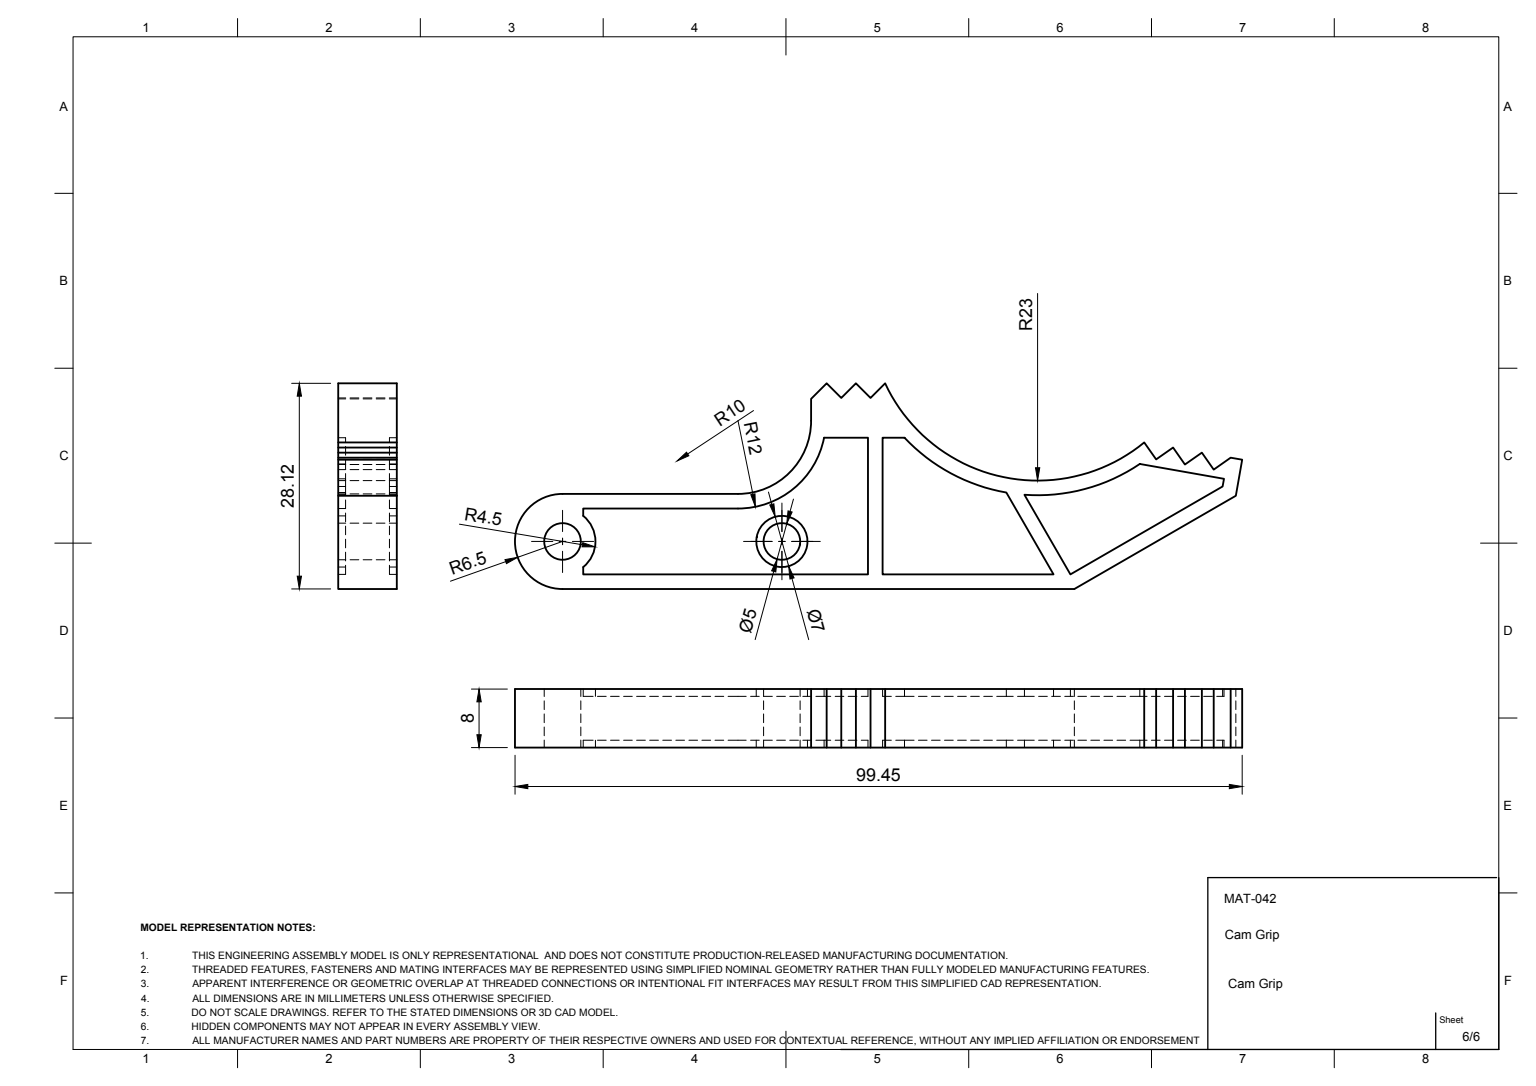
ISO-10303-21;
HEADER;
/* Generated by software containing ST-Developer
 * from STEP Tools, Inc. (www.steptools.com) 
 */

FILE_DESCRIPTION(
/* description */ ('STEP AP214'),
/* implementation_level */ '2;1');

FILE_NAME(
/* name */ 'Cam Grip.step',
/* time_stamp */ '2026-11-14T22:03:06-08:00',
/* author */ (''),
/* organization */ (''),
/* preprocessor_version */ 'ST-DEVELOPER v20.2',
/* originating_system */ 'Autodesk Translation Framework v15.17.0.0',
/* authorisation */ '');

FILE_SCHEMA (('AUTOMOTIVE_DESIGN { 1 0 10303 214 3 1 1 }'));
ENDSEC;

DATA;
#10=MECHANICAL_DESIGN_GEOMETRIC_PRESENTATION_REPRESENTATION('',(#308),#12966);
#288=SHAPE_REPRESENTATION_RELATIONSHIP('SRR','None',#13026,#296);
#296=ADVANCED_BREP_SHAPE_REPRESENTATION('',(#320),#12959);
#308=STYLED_ITEM('',(#13075),#320);
#320=MANIFOLD_SOLID_BREP('Body1',#5583);
#355=FACE_BOUND('',#953,.T.);
#356=FACE_BOUND('',#955,.T.);
#357=FACE_BOUND('',#957,.T.);
#358=FACE_BOUND('',#958,.T.);
#359=FACE_BOUND('',#959,.T.);
#360=FACE_BOUND('',#960,.T.);
#361=FACE_BOUND('',#962,.T.);
#362=FACE_BOUND('',#963,.T.);
#363=FACE_BOUND('',#964,.T.);
#364=FACE_BOUND('',#965,.T.);
#365=FACE_BOUND('',#1007,.T.);
#366=FACE_BOUND('',#1016,.T.);
#425=PLANE('',#5799);
#426=PLANE('',#5800);
#427=PLANE('',#5801);
#428=PLANE('',#5809);
#429=PLANE('',#5816);
#430=PLANE('',#5817);
#431=PLANE('',#5819);
#432=PLANE('',#5821);
#433=PLANE('',#5822);
#434=PLANE('',#5823);
#435=PLANE('',#5824);
#436=PLANE('',#5825);
#437=PLANE('',#5826);
#438=PLANE('',#5828);
#439=PLANE('',#5829);
#440=PLANE('',#5830);
#441=PLANE('',#5831);
#442=PLANE('',#5832);
#443=PLANE('',#5833);
#444=PLANE('',#5834);
#445=PLANE('',#5835);
#446=PLANE('',#5836);
#447=PLANE('',#5837);
#448=PLANE('',#5838);
#449=PLANE('',#5839);
#450=PLANE('',#5842);
#451=PLANE('',#5843);
#452=PLANE('',#5844);
#453=PLANE('',#5845);
#454=PLANE('',#5848);
#455=PLANE('',#5849);
#456=PLANE('',#5852);
#457=PLANE('',#5853);
#458=PLANE('',#5854);
#459=PLANE('',#5855);
#460=PLANE('',#5858);
#461=PLANE('',#5859);
#462=PLANE('',#5860);
#463=PLANE('',#5861);
#464=PLANE('',#5862);
#465=PLANE('',#5865);
#466=PLANE('',#5866);
#467=PLANE('',#5867);
#468=PLANE('',#5868);
#469=PLANE('',#5869);
#470=PLANE('',#5870);
#471=PLANE('',#5871);
#472=PLANE('',#5874);
#473=PLANE('',#5875);
#474=PLANE('',#5876);
#475=PLANE('',#5877);
#476=PLANE('',#5878);
#477=PLANE('',#5879);
#478=PLANE('',#5882);
#479=PLANE('',#5883);
#608=FACE_OUTER_BOUND('',#947,.T.);
#609=FACE_OUTER_BOUND('',#948,.T.);
#610=FACE_OUTER_BOUND('',#949,.T.);
#611=FACE_OUTER_BOUND('',#950,.T.);
#612=FACE_OUTER_BOUND('',#951,.T.);
#613=FACE_OUTER_BOUND('',#952,.T.);
#614=FACE_OUTER_BOUND('',#954,.T.);
#615=FACE_OUTER_BOUND('',#956,.T.);
#616=FACE_OUTER_BOUND('',#961,.T.);
#617=FACE_OUTER_BOUND('',#966,.T.);
#618=FACE_OUTER_BOUND('',#967,.T.);
#619=FACE_OUTER_BOUND('',#968,.T.);
#620=FACE_OUTER_BOUND('',#969,.T.);
#621=FACE_OUTER_BOUND('',#970,.T.);
#622=FACE_OUTER_BOUND('',#971,.T.);
#623=FACE_OUTER_BOUND('',#972,.T.);
#624=FACE_OUTER_BOUND('',#973,.T.);
#625=FACE_OUTER_BOUND('',#974,.T.);
#626=FACE_OUTER_BOUND('',#975,.T.);
#627=FACE_OUTER_BOUND('',#976,.T.);
#628=FACE_OUTER_BOUND('',#977,.T.);
#629=FACE_OUTER_BOUND('',#978,.T.);
#630=FACE_OUTER_BOUND('',#979,.T.);
#631=FACE_OUTER_BOUND('',#980,.T.);
#632=FACE_OUTER_BOUND('',#981,.T.);
#633=FACE_OUTER_BOUND('',#982,.T.);
#634=FACE_OUTER_BOUND('',#983,.T.);
#635=FACE_OUTER_BOUND('',#984,.T.);
#636=FACE_OUTER_BOUND('',#985,.T.);
#637=FACE_OUTER_BOUND('',#986,.T.);
#638=FACE_OUTER_BOUND('',#987,.T.);
#639=FACE_OUTER_BOUND('',#988,.T.);
#640=FACE_OUTER_BOUND('',#989,.T.);
#641=FACE_OUTER_BOUND('',#990,.T.);
#642=FACE_OUTER_BOUND('',#991,.T.);
#643=FACE_OUTER_BOUND('',#992,.T.);
#644=FACE_OUTER_BOUND('',#993,.T.);
#645=FACE_OUTER_BOUND('',#994,.T.);
#646=FACE_OUTER_BOUND('',#995,.T.);
#647=FACE_OUTER_BOUND('',#996,.T.);
#648=FACE_OUTER_BOUND('',#997,.T.);
#649=FACE_OUTER_BOUND('',#998,.T.);
#650=FACE_OUTER_BOUND('',#999,.T.);
#651=FACE_OUTER_BOUND('',#1000,.T.);
#652=FACE_OUTER_BOUND('',#1001,.T.);
#653=FACE_OUTER_BOUND('',#1002,.T.);
#654=FACE_OUTER_BOUND('',#1003,.T.);
#655=FACE_OUTER_BOUND('',#1004,.T.);
#656=FACE_OUTER_BOUND('',#1005,.T.);
#657=FACE_OUTER_BOUND('',#1006,.T.);
#658=FACE_OUTER_BOUND('',#1008,.T.);
#659=FACE_OUTER_BOUND('',#1009,.T.);
#660=FACE_OUTER_BOUND('',#1010,.T.);
#661=FACE_OUTER_BOUND('',#1011,.T.);
#662=FACE_OUTER_BOUND('',#1012,.T.);
#663=FACE_OUTER_BOUND('',#1013,.T.);
#664=FACE_OUTER_BOUND('',#1014,.T.);
#665=FACE_OUTER_BOUND('',#1015,.T.);
#666=FACE_OUTER_BOUND('',#1017,.T.);
#667=FACE_OUTER_BOUND('',#1018,.T.);
#668=FACE_OUTER_BOUND('',#1019,.T.);
#669=FACE_OUTER_BOUND('',#1020,.T.);
#670=FACE_OUTER_BOUND('',#1021,.T.);
#671=FACE_OUTER_BOUND('',#1022,.T.);
#672=FACE_OUTER_BOUND('',#1023,.T.);
#673=FACE_OUTER_BOUND('',#1024,.T.);
#674=FACE_OUTER_BOUND('',#1025,.T.);
#675=FACE_OUTER_BOUND('',#1026,.T.);
#676=FACE_OUTER_BOUND('',#1027,.T.);
#677=FACE_OUTER_BOUND('',#1028,.T.);
#947=EDGE_LOOP('',(#3931,#3932,#3933,#3934));
#948=EDGE_LOOP('',(#3935,#3936,#3937,#3938));
#949=EDGE_LOOP('',(#3939,#3940,#3941,#3942));
#950=EDGE_LOOP('',(#3943,#3944,#3945,#3946));
#951=EDGE_LOOP('',(#3947,#3948,#3949,#3950));
#952=EDGE_LOOP('',(#3951));
#953=EDGE_LOOP('',(#3952));
#954=EDGE_LOOP('',(#3953));
#955=EDGE_LOOP('',(#3954));
#956=EDGE_LOOP('',(#3955,#3956,#3957,#3958,#3959,#3960,#3961,#3962,#3963,
#3964,#3965,#3966,#3967,#3968,#3969,#3970,#3971,#3972,#3973,#3974));
#957=EDGE_LOOP('',(#3975,#3976,#3977,#3978,#3979,#3980,#3981,#3982));
#958=EDGE_LOOP('',(#3983,#3984,#3985,#3986,#3987));
#959=EDGE_LOOP('',(#3988,#3989,#3990,#3991,#3992));
#960=EDGE_LOOP('',(#3993));
#961=EDGE_LOOP('',(#3994,#3995,#3996,#3997,#3998,#3999,#4000,#4001,#4002,
#4003,#4004,#4005,#4006,#4007,#4008,#4009,#4010,#4011,#4012,#4013));
#962=EDGE_LOOP('',(#4014,#4015,#4016,#4017,#4018));
#963=EDGE_LOOP('',(#4019,#4020,#4021,#4022,#4023));
#964=EDGE_LOOP('',(#4024,#4025,#4026,#4027,#4028,#4029,#4030,#4031));
#965=EDGE_LOOP('',(#4032));
#966=EDGE_LOOP('',(#4033,#4034,#4035,#4036));
#967=EDGE_LOOP('',(#4037,#4038,#4039,#4040));
#968=EDGE_LOOP('',(#4041,#4042,#4043,#4044));
#969=EDGE_LOOP('',(#4045,#4046,#4047,#4048));
#970=EDGE_LOOP('',(#4049,#4050,#4051,#4052));
#971=EDGE_LOOP('',(#4053,#4054,#4055,#4056));
#972=EDGE_LOOP('',(#4057,#4058,#4059,#4060));
#973=EDGE_LOOP('',(#4061,#4062,#4063,#4064));
#974=EDGE_LOOP('',(#4065,#4066,#4067,#4068));
#975=EDGE_LOOP('',(#4069,#4070,#4071,#4072));
#976=EDGE_LOOP('',(#4073,#4074,#4075,#4076));
#977=EDGE_LOOP('',(#4077,#4078,#4079,#4080));
#978=EDGE_LOOP('',(#4081,#4082,#4083,#4084));
#979=EDGE_LOOP('',(#4085,#4086,#4087,#4088));
#980=EDGE_LOOP('',(#4089,#4090,#4091,#4092));
#981=EDGE_LOOP('',(#4093,#4094,#4095,#4096));
#982=EDGE_LOOP('',(#4097,#4098,#4099,#4100));
#983=EDGE_LOOP('',(#4101,#4102,#4103,#4104));
#984=EDGE_LOOP('',(#4105,#4106,#4107,#4108));
#985=EDGE_LOOP('',(#4109,#4110,#4111,#4112));
#986=EDGE_LOOP('',(#4113,#4114,#4115,#4116));
#987=EDGE_LOOP('',(#4117,#4118,#4119,#4120));
#988=EDGE_LOOP('',(#4121,#4122,#4123,#4124));
#989=EDGE_LOOP('',(#4125,#4126,#4127,#4128));
#990=EDGE_LOOP('',(#4129,#4130,#4131,#4132));
#991=EDGE_LOOP('',(#4133,#4134,#4135,#4136,#4137));
#992=EDGE_LOOP('',(#4138,#4139,#4140,#4141));
#993=EDGE_LOOP('',(#4142,#4143,#4144,#4145));
#994=EDGE_LOOP('',(#4146,#4147,#4148,#4149));
#995=EDGE_LOOP('',(#4150,#4151,#4152,#4153));
#996=EDGE_LOOP('',(#4154,#4155,#4156,#4157));
#997=EDGE_LOOP('',(#4158,#4159,#4160,#4161,#4162));
#998=EDGE_LOOP('',(#4163,#4164,#4165,#4166));
#999=EDGE_LOOP('',(#4167,#4168,#4169,#4170));
#1000=EDGE_LOOP('',(#4171,#4172,#4173,#4174));
#1001=EDGE_LOOP('',(#4175,#4176,#4177,#4178));
#1002=EDGE_LOOP('',(#4179,#4180,#4181,#4182));
#1003=EDGE_LOOP('',(#4183,#4184,#4185,#4186));
#1004=EDGE_LOOP('',(#4187,#4188,#4189,#4190));
#1005=EDGE_LOOP('',(#4191,#4192,#4193,#4194));
#1006=EDGE_LOOP('',(#4195,#4196,#4197,#4198,#4199,#4200,#4201,#4202));
#1007=EDGE_LOOP('',(#4203));
#1008=EDGE_LOOP('',(#4204,#4205,#4206,#4207));
#1009=EDGE_LOOP('',(#4208,#4209,#4210,#4211));
#1010=EDGE_LOOP('',(#4212,#4213,#4214,#4215));
#1011=EDGE_LOOP('',(#4216,#4217,#4218,#4219));
#1012=EDGE_LOOP('',(#4220,#4221,#4222,#4223));
#1013=EDGE_LOOP('',(#4224,#4225,#4226,#4227));
#1014=EDGE_LOOP('',(#4228,#4229,#4230,#4231));
#1015=EDGE_LOOP('',(#4232,#4233,#4234,#4235,#4236,#4237,#4238,#4239));
#1016=EDGE_LOOP('',(#4240));
#1017=EDGE_LOOP('',(#4241,#4242,#4243,#4244));
#1018=EDGE_LOOP('',(#4245,#4246,#4247,#4248));
#1019=EDGE_LOOP('',(#4249,#4250,#4251,#4252));
#1020=EDGE_LOOP('',(#4253,#4254,#4255,#4256));
#1021=EDGE_LOOP('',(#4257,#4258,#4259,#4260));
#1022=EDGE_LOOP('',(#4261,#4262,#4263,#4264,#4265));
#1023=EDGE_LOOP('',(#4266,#4267,#4268,#4269));
#1024=EDGE_LOOP('',(#4270,#4271,#4272,#4273));
#1025=EDGE_LOOP('',(#4274,#4275,#4276,#4277));
#1026=EDGE_LOOP('',(#4278,#4279,#4280,#4281));
#1027=EDGE_LOOP('',(#4282,#4283,#4284,#4285));
#1028=EDGE_LOOP('',(#4286,#4287,#4288,#4289,#4290));
#1334=LINE('',#8070,#1791);
#1335=LINE('',#8077,#1792);
#1336=LINE('',#8080,#1793);
#1337=LINE('',#8085,#1794);
#1338=LINE('',#8091,#1795);
#1339=LINE('',#8097,#1796);
#1340=LINE('',#8104,#1797);
#1341=LINE('',#8106,#1798);
#1342=LINE('',#8110,#1799);
#1343=LINE('',#8114,#1800);
#1344=LINE('',#8116,#1801);
#1345=LINE('',#8118,#1802);
#1346=LINE('',#8120,#1803);
#1347=LINE('',#8122,#1804);
#1348=LINE('',#8124,#1805);
#1349=LINE('',#8128,#1806);
#1350=LINE('',#8130,#1807);
#1351=LINE('',#8132,#1808);
#1352=LINE('',#8134,#1809);
#1353=LINE('',#8136,#1810);
#1354=LINE('',#8138,#1811);
#1355=LINE('',#8140,#1812);
#1356=LINE('',#8141,#1813);
#1357=LINE('',#8146,#1814);
#1358=LINE('',#8148,#1815);
#1359=LINE('',#8150,#1816);
#1360=LINE('',#8152,#1817);
#1361=LINE('',#8156,#1818);
#1362=LINE('',#8157,#1819);
#1363=LINE('',#8160,#1820);
#1364=LINE('',#8162,#1821);
#1365=LINE('',#8164,#1822);
#1366=LINE('',#8167,#1823);
#1367=LINE('',#8170,#1824);
#1368=LINE('',#8172,#1825);
#1369=LINE('',#8174,#1826);
#1370=LINE('',#8176,#1827);
#1371=LINE('',#8181,#1828);
#1372=LINE('',#8183,#1829);
#1373=LINE('',#8185,#1830);
#1374=LINE('',#8187,#1831);
#1375=LINE('',#8189,#1832);
#1376=LINE('',#8191,#1833);
#1377=LINE('',#8193,#1834);
#1378=LINE('',#8195,#1835);
#1379=LINE('',#8197,#1836);
#1380=LINE('',#8201,#1837);
#1381=LINE('',#8203,#1838);
#1382=LINE('',#8205,#1839);
#1383=LINE('',#8207,#1840);
#1384=LINE('',#8209,#1841);
#1385=LINE('',#8211,#1842);
#1386=LINE('',#8215,#1843);
#1387=LINE('',#8218,#1844);
#1388=LINE('',#8221,#1845);
#1389=LINE('',#8223,#1846);
#1390=LINE('',#8225,#1847);
#1391=LINE('',#8227,#1848);
#1392=LINE('',#8231,#1849);
#1393=LINE('',#8233,#1850);
#1394=LINE('',#8235,#1851);
#1395=LINE('',#8238,#1852);
#1396=LINE('',#8240,#1853);
#1397=LINE('',#8242,#1854);
#1398=LINE('',#8246,#1855);
#1399=LINE('',#8248,#1856);
#1400=LINE('',#8250,#1857);
#1401=LINE('',#8251,#1858);
#1402=LINE('',#8253,#1859);
#1403=LINE('',#8254,#1860);
#1404=LINE('',#8256,#1861);
#1405=LINE('',#8258,#1862);
#1406=LINE('',#8260,#1863);
#1407=LINE('',#8262,#1864);
#1408=LINE('',#8264,#1865);
#1409=LINE('',#8266,#1866);
#1410=LINE('',#8268,#1867);
#1411=LINE('',#8270,#1868);
#1412=LINE('',#8272,#1869);
#1413=LINE('',#8274,#1870);
#1414=LINE('',#8276,#1871);
#1415=LINE('',#8278,#1872);
#1416=LINE('',#8280,#1873);
#1417=LINE('',#8282,#1874);
#1418=LINE('',#8284,#1875);
#1419=LINE('',#8286,#1876);
#1420=LINE('',#8288,#1877);
#1421=LINE('',#8290,#1878);
#1422=LINE('',#8294,#1879);
#1423=LINE('',#8296,#1880);
#1424=LINE('',#8297,#1881);
#1425=LINE('',#8300,#1882);
#1426=LINE('',#8301,#1883);
#1427=LINE('',#8304,#1884);
#1428=LINE('',#8305,#1885);
#1429=LINE('',#8308,#1886);
#1430=LINE('',#8309,#1887);
#1431=LINE('',#8315,#1888);
#1432=LINE('',#8317,#1889);
#1433=LINE('',#8318,#1890);
#1434=LINE('',#8321,#1891);
#1435=LINE('',#8322,#1892);
#1436=LINE('',#8325,#1893);
#1437=LINE('',#8326,#1894);
#1438=LINE('',#8330,#1895);
#1439=LINE('',#8332,#1896);
#1440=LINE('',#8336,#1897);
#1441=LINE('',#8339,#1898);
#1442=LINE('',#8342,#1899);
#1443=LINE('',#8343,#1900);
#1444=LINE('',#8346,#1901);
#1445=LINE('',#8347,#1902);
#1446=LINE('',#8350,#1903);
#1447=LINE('',#8351,#1904);
#1448=LINE('',#8354,#1905);
#1449=LINE('',#8355,#1906);
#1450=LINE('',#8359,#1907);
#1451=LINE('',#8362,#1908);
#1452=LINE('',#8363,#1909);
#1453=LINE('',#8365,#1910);
#1454=LINE('',#8369,#1911);
#1455=LINE('',#8370,#1912);
#1456=LINE('',#8373,#1913);
#1457=LINE('',#8374,#1914);
#1458=LINE('',#8378,#1915);
#1459=LINE('',#8381,#1916);
#1460=LINE('',#8382,#1917);
#1461=LINE('',#8385,#1918);
#1462=LINE('',#8386,#1919);
#1463=LINE('',#8389,#1920);
#1464=LINE('',#8390,#1921);
#1465=LINE('',#8392,#1922);
#1466=LINE('',#8396,#1923);
#1467=LINE('',#8398,#1924);
#1468=LINE('',#8399,#1925);
#1469=LINE('',#8402,#1926);
#1470=LINE('',#8403,#1927);
#1471=LINE('',#8407,#1928);
#1472=LINE('',#8410,#1929);
#1473=LINE('',#8411,#1930);
#1474=LINE('',#8413,#1931);
#1475=LINE('',#8417,#1932);
#1476=LINE('',#8419,#1933);
#1477=LINE('',#8420,#1934);
#1478=LINE('',#8423,#1935);
#1479=LINE('',#8424,#1936);
#1480=LINE('',#8427,#1937);
#1481=LINE('',#8428,#1938);
#1482=LINE('',#8432,#1939);
#1483=LINE('',#8434,#1940);
#1791=VECTOR('',#6536,3.5);
#1792=VECTOR('',#6543,1000.);
#1793=VECTOR('',#6546,1000.);
#1794=VECTOR('',#6551,3.5);
#1795=VECTOR('',#6558,2.5);
#1796=VECTOR('',#6565,2.5);
#1797=VECTOR('',#6574,1000.);
#1798=VECTOR('',#6575,1000.);
#1799=VECTOR('',#6578,1000.);
#1800=VECTOR('',#6581,1000.);
#1801=VECTOR('',#6582,1000.);
#1802=VECTOR('',#6583,1000.);
#1803=VECTOR('',#6584,1000.);
#1804=VECTOR('',#6585,1000.);
#1805=VECTOR('',#6586,1000.);
#1806=VECTOR('',#6589,1000.);
#1807=VECTOR('',#6590,1000.);
#1808=VECTOR('',#6591,1000.);
#1809=VECTOR('',#6592,1000.);
#1810=VECTOR('',#6593,1000.);
#1811=VECTOR('',#6594,1000.);
#1812=VECTOR('',#6595,1000.);
#1813=VECTOR('',#6596,1000.);
#1814=VECTOR('',#6599,1000.);
#1815=VECTOR('',#6600,1000.);
#1816=VECTOR('',#6601,1000.);
#1817=VECTOR('',#6602,1000.);
#1818=VECTOR('',#6605,1000.);
#1819=VECTOR('',#6606,1000.);
#1820=VECTOR('',#6607,1000.);
#1821=VECTOR('',#6608,1000.);
#1822=VECTOR('',#6609,1000.);
#1823=VECTOR('',#6612,1000.);
#1824=VECTOR('',#6613,1000.);
#1825=VECTOR('',#6614,1000.);
#1826=VECTOR('',#6615,1000.);
#1827=VECTOR('',#6616,1000.);
#1828=VECTOR('',#6621,1000.);
#1829=VECTOR('',#6622,1000.);
#1830=VECTOR('',#6623,1000.);
#1831=VECTOR('',#6624,1000.);
#1832=VECTOR('',#6625,1000.);
#1833=VECTOR('',#6626,1000.);
#1834=VECTOR('',#6627,1000.);
#1835=VECTOR('',#6628,1000.);
#1836=VECTOR('',#6629,1000.);
#1837=VECTOR('',#6632,1000.);
#1838=VECTOR('',#6633,1000.);
#1839=VECTOR('',#6634,1000.);
#1840=VECTOR('',#6635,1000.);
#1841=VECTOR('',#6636,1000.);
#1842=VECTOR('',#6637,1000.);
#1843=VECTOR('',#6640,1000.);
#1844=VECTOR('',#6643,1000.);
#1845=VECTOR('',#6644,1000.);
#1846=VECTOR('',#6645,1000.);
#1847=VECTOR('',#6646,1000.);
#1848=VECTOR('',#6647,1000.);
#1849=VECTOR('',#6650,1000.);
#1850=VECTOR('',#6651,1000.);
#1851=VECTOR('',#6652,1000.);
#1852=VECTOR('',#6655,1000.);
#1853=VECTOR('',#6656,1000.);
#1854=VECTOR('',#6657,1000.);
#1855=VECTOR('',#6660,1000.);
#1856=VECTOR('',#6661,1000.);
#1857=VECTOR('',#6662,1000.);
#1858=VECTOR('',#6663,1000.);
#1859=VECTOR('',#6666,1000.);
#1860=VECTOR('',#6667,1000.);
#1861=VECTOR('',#6670,1000.);
#1862=VECTOR('',#6673,1000.);
#1863=VECTOR('',#6676,1000.);
#1864=VECTOR('',#6679,1000.);
#1865=VECTOR('',#6682,1000.);
#1866=VECTOR('',#6685,1000.);
#1867=VECTOR('',#6688,1000.);
#1868=VECTOR('',#6691,1000.);
#1869=VECTOR('',#6694,1000.);
#1870=VECTOR('',#6697,1000.);
#1871=VECTOR('',#6700,1000.);
#1872=VECTOR('',#6703,1000.);
#1873=VECTOR('',#6706,1000.);
#1874=VECTOR('',#6709,1000.);
#1875=VECTOR('',#6712,1000.);
#1876=VECTOR('',#6715,1000.);
#1877=VECTOR('',#6718,1000.);
#1878=VECTOR('',#6721,1000.);
#1879=VECTOR('',#6726,1000.);
#1880=VECTOR('',#6727,1000.);
#1881=VECTOR('',#6728,1000.);
#1882=VECTOR('',#6731,1000.);
#1883=VECTOR('',#6732,1000.);
#1884=VECTOR('',#6735,1000.);
#1885=VECTOR('',#6736,1000.);
#1886=VECTOR('',#6739,1000.);
#1887=VECTOR('',#6740,1000.);
#1888=VECTOR('',#6749,1000.);
#1889=VECTOR('',#6750,1000.);
#1890=VECTOR('',#6751,1000.);
#1891=VECTOR('',#6754,1000.);
#1892=VECTOR('',#6755,1000.);
#1893=VECTOR('',#6758,1000.);
#1894=VECTOR('',#6759,1000.);
#1895=VECTOR('',#6764,1000.);
#1896=VECTOR('',#6767,1000.);
#1897=VECTOR('',#6772,1000.);
#1898=VECTOR('',#6775,1000.);
#1899=VECTOR('',#6778,1000.);
#1900=VECTOR('',#6779,1000.);
#1901=VECTOR('',#6782,1000.);
#1902=VECTOR('',#6783,1000.);
#1903=VECTOR('',#6786,1000.);
#1904=VECTOR('',#6787,1000.);
#1905=VECTOR('',#6790,1000.);
#1906=VECTOR('',#6791,1000.);
#1907=VECTOR('',#6796,1000.);
#1908=VECTOR('',#6799,1000.);
#1909=VECTOR('',#6800,1000.);
#1910=VECTOR('',#6803,1000.);
#1911=VECTOR('',#6808,1000.);
#1912=VECTOR('',#6809,1000.);
#1913=VECTOR('',#6812,1000.);
#1914=VECTOR('',#6813,1000.);
#1915=VECTOR('',#6818,1000.);
#1916=VECTOR('',#6821,1000.);
#1917=VECTOR('',#6822,1000.);
#1918=VECTOR('',#6825,1000.);
#1919=VECTOR('',#6826,1000.);
#1920=VECTOR('',#6829,1000.);
#1921=VECTOR('',#6830,1000.);
#1922=VECTOR('',#6833,1000.);
#1923=VECTOR('',#6838,1000.);
#1924=VECTOR('',#6839,1000.);
#1925=VECTOR('',#6840,1000.);
#1926=VECTOR('',#6843,1000.);
#1927=VECTOR('',#6844,1000.);
#1928=VECTOR('',#6849,1000.);
#1929=VECTOR('',#6852,1000.);
#1930=VECTOR('',#6853,1000.);
#1931=VECTOR('',#6856,1000.);
#1932=VECTOR('',#6861,1000.);
#1933=VECTOR('',#6862,1000.);
#1934=VECTOR('',#6863,1000.);
#1935=VECTOR('',#6866,1000.);
#1936=VECTOR('',#6867,1000.);
#1937=VECTOR('',#6870,1000.);
#1938=VECTOR('',#6871,1000.);
#1939=VECTOR('',#6876,1000.);
#1940=VECTOR('',#6879,1000.);
#2192=CIRCLE('',#5785,3.5);
#2193=CIRCLE('',#5786,3.5);
#2194=CIRCLE('',#5788,4.5);
#2195=CIRCLE('',#5789,4.5);
#2196=CIRCLE('',#5791,3.5);
#2197=CIRCLE('',#5792,3.5);
#2198=CIRCLE('',#5794,2.5);
#2199=CIRCLE('',#5795,2.5);
#2200=CIRCLE('',#5797,2.5);
#2201=CIRCLE('',#5798,2.5);
#2202=CIRCLE('',#5802,6.50000000000001);
#2203=CIRCLE('',#5803,10.);
#2204=CIRCLE('',#5804,22.9999999999999);
#2205=CIRCLE('',#5805,4.5);
#2206=CIRCLE('',#5806,12.);
#2207=CIRCLE('',#5807,24.9999999999999);
#2208=CIRCLE('',#5808,24.9999999999999);
#2209=CIRCLE('',#5810,22.9999999999999);
#2210=CIRCLE('',#5811,10.);
#2211=CIRCLE('',#5812,6.50000000000001);
#2212=CIRCLE('',#5813,24.9999999999999);
#2213=CIRCLE('',#5814,24.9999999999999);
#2214=CIRCLE('',#5815,12.);
#2215=CIRCLE('',#5841,24.9999999999999);
#2216=CIRCLE('',#5847,24.9999999999999);
#2217=CIRCLE('',#5851,4.5);
#2218=CIRCLE('',#5857,12.);
#2219=CIRCLE('',#5864,12.);
#2220=CIRCLE('',#5873,24.9999999999999);
#2221=CIRCLE('',#5881,24.9999999999999);
#2472=VERTEX_POINT('',#8067);
#2473=VERTEX_POINT('',#8069);
#2474=VERTEX_POINT('',#8073);
#2475=VERTEX_POINT('',#8074);
#2476=VERTEX_POINT('',#8076);
#2477=VERTEX_POINT('',#8078);
#2478=VERTEX_POINT('',#8082);
#2479=VERTEX_POINT('',#8084);
#2480=VERTEX_POINT('',#8088);
#2481=VERTEX_POINT('',#8090);
#2482=VERTEX_POINT('',#8094);
#2483=VERTEX_POINT('',#8096);
#2484=VERTEX_POINT('',#8102);
#2485=VERTEX_POINT('',#8103);
#2486=VERTEX_POINT('',#8105);
#2487=VERTEX_POINT('',#8107);
#2488=VERTEX_POINT('',#8109);
#2489=VERTEX_POINT('',#8111);
#2490=VERTEX_POINT('',#8113);
#2491=VERTEX_POINT('',#8115);
#2492=VERTEX_POINT('',#8117);
#2493=VERTEX_POINT('',#8119);
#2494=VERTEX_POINT('',#8121);
#2495=VERTEX_POINT('',#8123);
#2496=VERTEX_POINT('',#8125);
#2497=VERTEX_POINT('',#8127);
#2498=VERTEX_POINT('',#8129);
#2499=VERTEX_POINT('',#8131);
#2500=VERTEX_POINT('',#8133);
#2501=VERTEX_POINT('',#8135);
#2502=VERTEX_POINT('',#8137);
#2503=VERTEX_POINT('',#8139);
#2504=VERTEX_POINT('',#8142);
#2505=VERTEX_POINT('',#8143);
#2506=VERTEX_POINT('',#8145);
#2507=VERTEX_POINT('',#8147);
#2508=VERTEX_POINT('',#8149);
#2509=VERTEX_POINT('',#8151);
#2510=VERTEX_POINT('',#8153);
#2511=VERTEX_POINT('',#8155);
#2512=VERTEX_POINT('',#8158);
#2513=VERTEX_POINT('',#8159);
#2514=VERTEX_POINT('',#8161);
#2515=VERTEX_POINT('',#8163);
#2516=VERTEX_POINT('',#8165);
#2517=VERTEX_POINT('',#8168);
#2518=VERTEX_POINT('',#8169);
#2519=VERTEX_POINT('',#8171);
#2520=VERTEX_POINT('',#8173);
#2521=VERTEX_POINT('',#8175);
#2522=VERTEX_POINT('',#8179);
#2523=VERTEX_POINT('',#8180);
#2524=VERTEX_POINT('',#8182);
#2525=VERTEX_POINT('',#8184);
#2526=VERTEX_POINT('',#8186);
#2527=VERTEX_POINT('',#8188);
#2528=VERTEX_POINT('',#8190);
#2529=VERTEX_POINT('',#8192);
#2530=VERTEX_POINT('',#8194);
#2531=VERTEX_POINT('',#8196);
#2532=VERTEX_POINT('',#8198);
#2533=VERTEX_POINT('',#8200);
#2534=VERTEX_POINT('',#8202);
#2535=VERTEX_POINT('',#8204);
#2536=VERTEX_POINT('',#8206);
#2537=VERTEX_POINT('',#8208);
#2538=VERTEX_POINT('',#8210);
#2539=VERTEX_POINT('',#8212);
#2540=VERTEX_POINT('',#8214);
#2541=VERTEX_POINT('',#8216);
#2542=VERTEX_POINT('',#8219);
#2543=VERTEX_POINT('',#8220);
#2544=VERTEX_POINT('',#8222);
#2545=VERTEX_POINT('',#8224);
#2546=VERTEX_POINT('',#8226);
#2547=VERTEX_POINT('',#8229);
#2548=VERTEX_POINT('',#8230);
#2549=VERTEX_POINT('',#8232);
#2550=VERTEX_POINT('',#8234);
#2551=VERTEX_POINT('',#8236);
#2552=VERTEX_POINT('',#8239);
#2553=VERTEX_POINT('',#8241);
#2554=VERTEX_POINT('',#8243);
#2555=VERTEX_POINT('',#8245);
#2556=VERTEX_POINT('',#8247);
#2557=VERTEX_POINT('',#8249);
#2558=VERTEX_POINT('',#8293);
#2559=VERTEX_POINT('',#8295);
#2560=VERTEX_POINT('',#8299);
#2561=VERTEX_POINT('',#8303);
#2562=VERTEX_POINT('',#8307);
#2563=VERTEX_POINT('',#8314);
#2564=VERTEX_POINT('',#8316);
#2565=VERTEX_POINT('',#8320);
#2566=VERTEX_POINT('',#8324);
#2567=VERTEX_POINT('',#8328);
#2568=VERTEX_POINT('',#8335);
#2569=VERTEX_POINT('',#8337);
#2570=VERTEX_POINT('',#8341);
#2571=VERTEX_POINT('',#8345);
#2572=VERTEX_POINT('',#8349);
#2573=VERTEX_POINT('',#8353);
#2574=VERTEX_POINT('',#8357);
#2575=VERTEX_POINT('',#8361);
#2576=VERTEX_POINT('',#8368);
#2577=VERTEX_POINT('',#8372);
#2578=VERTEX_POINT('',#8376);
#2579=VERTEX_POINT('',#8380);
#2580=VERTEX_POINT('',#8384);
#2581=VERTEX_POINT('',#8388);
#2582=VERTEX_POINT('',#8395);
#2583=VERTEX_POINT('',#8397);
#2584=VERTEX_POINT('',#8401);
#2585=VERTEX_POINT('',#8405);
#2586=VERTEX_POINT('',#8409);
#2587=VERTEX_POINT('',#8416);
#2588=VERTEX_POINT('',#8418);
#2589=VERTEX_POINT('',#8422);
#2590=VERTEX_POINT('',#8426);
#2591=VERTEX_POINT('',#8430);
#3022=EDGE_CURVE('',#2472,#2472,#2192,.T.);
#3023=EDGE_CURVE('',#2472,#2473,#1334,.T.);
#3024=EDGE_CURVE('',#2473,#2473,#2193,.T.);
#3025=EDGE_CURVE('',#2474,#2475,#2194,.T.);
#3026=EDGE_CURVE('',#2474,#2476,#1335,.T.);
#3027=EDGE_CURVE('',#2476,#2477,#2195,.T.);
#3028=EDGE_CURVE('',#2475,#2477,#1336,.T.);
#3029=EDGE_CURVE('',#2478,#2478,#2196,.T.);
#3030=EDGE_CURVE('',#2478,#2479,#1337,.T.);
#3031=EDGE_CURVE('',#2479,#2479,#2197,.T.);
#3032=EDGE_CURVE('',#2480,#2480,#2198,.T.);
#3033=EDGE_CURVE('',#2480,#2481,#1338,.T.);
#3034=EDGE_CURVE('',#2481,#2481,#2199,.T.);
#3035=EDGE_CURVE('',#2482,#2482,#2200,.T.);
#3036=EDGE_CURVE('',#2482,#2483,#1339,.T.);
#3037=EDGE_CURVE('',#2483,#2483,#2201,.T.);
#3038=EDGE_CURVE('',#2484,#2485,#1340,.T.);
#3039=EDGE_CURVE('',#2485,#2486,#1341,.T.);
#3040=EDGE_CURVE('',#2486,#2487,#2202,.T.);
#3041=EDGE_CURVE('',#2487,#2488,#1342,.T.);
#3042=EDGE_CURVE('',#2488,#2489,#2203,.T.);
#3043=EDGE_CURVE('',#2489,#2490,#1343,.T.);
#3044=EDGE_CURVE('',#2490,#2491,#1344,.T.);
#3045=EDGE_CURVE('',#2491,#2492,#1345,.T.);
#3046=EDGE_CURVE('',#2492,#2493,#1346,.T.);
#3047=EDGE_CURVE('',#2493,#2494,#1347,.T.);
#3048=EDGE_CURVE('',#2494,#2495,#1348,.T.);
#3049=EDGE_CURVE('',#2495,#2496,#2204,.T.);
#3050=EDGE_CURVE('',#2496,#2497,#1349,.T.);
#3051=EDGE_CURVE('',#2497,#2498,#1350,.T.);
#3052=EDGE_CURVE('',#2498,#2499,#1351,.T.);
#3053=EDGE_CURVE('',#2499,#2500,#1352,.T.);
#3054=EDGE_CURVE('',#2500,#2501,#1353,.T.);
#3055=EDGE_CURVE('',#2501,#2502,#1354,.T.);
#3056=EDGE_CURVE('',#2502,#2503,#1355,.T.);
#3057=EDGE_CURVE('',#2503,#2484,#1356,.T.);
#3058=EDGE_CURVE('',#2504,#2505,#2205,.T.);
#3059=EDGE_CURVE('',#2506,#2504,#1357,.T.);
#3060=EDGE_CURVE('',#2507,#2506,#1358,.T.);
#3061=EDGE_CURVE('',#2508,#2507,#1359,.T.);
#3062=EDGE_CURVE('',#2509,#2508,#1360,.T.);
#3063=EDGE_CURVE('',#2510,#2509,#2206,.T.);
#3064=EDGE_CURVE('',#2511,#2510,#1361,.T.);
#3065=EDGE_CURVE('',#2505,#2511,#1362,.T.);
#3066=EDGE_CURVE('',#2512,#2513,#1363,.T.);
#3067=EDGE_CURVE('',#2514,#2512,#1364,.T.);
#3068=EDGE_CURVE('',#2515,#2514,#1365,.T.);
#3069=EDGE_CURVE('',#2516,#2515,#2207,.T.);
#3070=EDGE_CURVE('',#2513,#2516,#1366,.T.);
#3071=EDGE_CURVE('',#2517,#2518,#1367,.T.);
#3072=EDGE_CURVE('',#2519,#2517,#1368,.T.);
#3073=EDGE_CURVE('',#2520,#2519,#1369,.T.);
#3074=EDGE_CURVE('',#2521,#2520,#1370,.T.);
#3075=EDGE_CURVE('',#2518,#2521,#2208,.T.);
#3076=EDGE_CURVE('',#2522,#2523,#1371,.T.);
#3077=EDGE_CURVE('',#2524,#2522,#1372,.T.);
#3078=EDGE_CURVE('',#2525,#2524,#1373,.T.);
#3079=EDGE_CURVE('',#2526,#2525,#1374,.T.);
#3080=EDGE_CURVE('',#2527,#2526,#1375,.T.);
#3081=EDGE_CURVE('',#2528,#2527,#1376,.T.);
#3082=EDGE_CURVE('',#2529,#2528,#1377,.T.);
#3083=EDGE_CURVE('',#2530,#2529,#1378,.T.);
#3084=EDGE_CURVE('',#2531,#2530,#1379,.T.);
#3085=EDGE_CURVE('',#2532,#2531,#2209,.T.);
#3086=EDGE_CURVE('',#2533,#2532,#1380,.T.);
#3087=EDGE_CURVE('',#2534,#2533,#1381,.T.);
#3088=EDGE_CURVE('',#2535,#2534,#1382,.T.);
#3089=EDGE_CURVE('',#2536,#2535,#1383,.T.);
#3090=EDGE_CURVE('',#2537,#2536,#1384,.T.);
#3091=EDGE_CURVE('',#2538,#2537,#1385,.T.);
#3092=EDGE_CURVE('',#2539,#2538,#2210,.T.);
#3093=EDGE_CURVE('',#2540,#2539,#1386,.T.);
#3094=EDGE_CURVE('',#2541,#2540,#2211,.T.);
#3095=EDGE_CURVE('',#2523,#2541,#1387,.T.);
#3096=EDGE_CURVE('',#2542,#2543,#1388,.T.);
#3097=EDGE_CURVE('',#2544,#2542,#1389,.T.);
#3098=EDGE_CURVE('',#2545,#2544,#1390,.T.);
#3099=EDGE_CURVE('',#2546,#2545,#1391,.T.);
#3100=EDGE_CURVE('',#2543,#2546,#2212,.T.);
#3101=EDGE_CURVE('',#2547,#2548,#1392,.T.);
#3102=EDGE_CURVE('',#2549,#2547,#1393,.T.);
#3103=EDGE_CURVE('',#2550,#2549,#1394,.T.);
#3104=EDGE_CURVE('',#2551,#2550,#2213,.T.);
#3105=EDGE_CURVE('',#2548,#2551,#1395,.T.);
#3106=EDGE_CURVE('',#2552,#2476,#1396,.T.);
#3107=EDGE_CURVE('',#2553,#2552,#1397,.T.);
#3108=EDGE_CURVE('',#2554,#2553,#2214,.T.);
#3109=EDGE_CURVE('',#2555,#2554,#1398,.T.);
#3110=EDGE_CURVE('',#2556,#2555,#1399,.T.);
#3111=EDGE_CURVE('',#2557,#2556,#1400,.T.);
#3112=EDGE_CURVE('',#2477,#2557,#1401,.T.);
#3113=EDGE_CURVE('',#2485,#2523,#1402,.T.);
#3114=EDGE_CURVE('',#2484,#2522,#1403,.T.);
#3115=EDGE_CURVE('',#2486,#2541,#1404,.T.);
#3116=EDGE_CURVE('',#2487,#2540,#1405,.T.);
#3117=EDGE_CURVE('',#2488,#2539,#1406,.T.);
#3118=EDGE_CURVE('',#2489,#2538,#1407,.T.);
#3119=EDGE_CURVE('',#2490,#2537,#1408,.T.);
#3120=EDGE_CURVE('',#2491,#2536,#1409,.T.);
#3121=EDGE_CURVE('',#2492,#2535,#1410,.T.);
#3122=EDGE_CURVE('',#2493,#2534,#1411,.T.);
#3123=EDGE_CURVE('',#2494,#2533,#1412,.T.);
#3124=EDGE_CURVE('',#2495,#2532,#1413,.T.);
#3125=EDGE_CURVE('',#2496,#2531,#1414,.T.);
#3126=EDGE_CURVE('',#2497,#2530,#1415,.T.);
#3127=EDGE_CURVE('',#2498,#2529,#1416,.T.);
#3128=EDGE_CURVE('',#2499,#2528,#1417,.T.);
#3129=EDGE_CURVE('',#2500,#2527,#1418,.T.);
#3130=EDGE_CURVE('',#2501,#2526,#1419,.T.);
#3131=EDGE_CURVE('',#2502,#2525,#1420,.T.);
#3132=EDGE_CURVE('',#2503,#2524,#1421,.T.);
#3133=EDGE_CURVE('',#2558,#2518,#1422,.T.);
#3134=EDGE_CURVE('',#2559,#2558,#1423,.T.);
#3135=EDGE_CURVE('',#2559,#2517,#1424,.T.);
#3136=EDGE_CURVE('',#2560,#2559,#1425,.T.);
#3137=EDGE_CURVE('',#2560,#2519,#1426,.T.);
#3138=EDGE_CURVE('',#2561,#2560,#1427,.T.);
#3139=EDGE_CURVE('',#2561,#2520,#1428,.T.);
#3140=EDGE_CURVE('',#2562,#2561,#1429,.T.);
#3141=EDGE_CURVE('',#2562,#2521,#1430,.T.);
#3142=EDGE_CURVE('',#2558,#2562,#2215,.T.);
#3143=EDGE_CURVE('',#2563,#2513,#1431,.T.);
#3144=EDGE_CURVE('',#2564,#2563,#1432,.T.);
#3145=EDGE_CURVE('',#2564,#2512,#1433,.T.);
#3146=EDGE_CURVE('',#2565,#2564,#1434,.T.);
#3147=EDGE_CURVE('',#2565,#2514,#1435,.T.);
#3148=EDGE_CURVE('',#2566,#2565,#1436,.T.);
#3149=EDGE_CURVE('',#2566,#2515,#1437,.T.);
#3150=EDGE_CURVE('',#2567,#2566,#2216,.T.);
#3151=EDGE_CURVE('',#2567,#2516,#1438,.T.);
#3152=EDGE_CURVE('',#2563,#2567,#1439,.T.);
#3153=EDGE_CURVE('',#2568,#2505,#1440,.T.);
#3154=EDGE_CURVE('',#2569,#2568,#2217,.T.);
#3155=EDGE_CURVE('',#2569,#2504,#1441,.T.);
#3156=EDGE_CURVE('',#2570,#2569,#1442,.T.);
#3157=EDGE_CURVE('',#2570,#2506,#1443,.T.);
#3158=EDGE_CURVE('',#2571,#2570,#1444,.T.);
#3159=EDGE_CURVE('',#2571,#2507,#1445,.T.);
#3160=EDGE_CURVE('',#2572,#2571,#1446,.T.);
#3161=EDGE_CURVE('',#2572,#2508,#1447,.T.);
#3162=EDGE_CURVE('',#2573,#2572,#1448,.T.);
#3163=EDGE_CURVE('',#2573,#2509,#1449,.T.);
#3164=EDGE_CURVE('',#2574,#2573,#2218,.T.);
#3165=EDGE_CURVE('',#2574,#2510,#1450,.T.);
#3166=EDGE_CURVE('',#2575,#2574,#1451,.T.);
#3167=EDGE_CURVE('',#2575,#2511,#1452,.T.);
#3168=EDGE_CURVE('',#2568,#2575,#1453,.T.);
#3169=EDGE_CURVE('',#2576,#2474,#1454,.T.);
#3170=EDGE_CURVE('',#2576,#2552,#1455,.T.);
#3171=EDGE_CURVE('',#2577,#2576,#1456,.T.);
#3172=EDGE_CURVE('',#2577,#2553,#1457,.T.);
#3173=EDGE_CURVE('',#2578,#2577,#2219,.T.);
#3174=EDGE_CURVE('',#2578,#2554,#1458,.T.);
#3175=EDGE_CURVE('',#2579,#2578,#1459,.T.);
#3176=EDGE_CURVE('',#2579,#2555,#1460,.T.);
#3177=EDGE_CURVE('',#2580,#2579,#1461,.T.);
#3178=EDGE_CURVE('',#2580,#2556,#1462,.T.);
#3179=EDGE_CURVE('',#2581,#2580,#1463,.T.);
#3180=EDGE_CURVE('',#2581,#2557,#1464,.T.);
#3181=EDGE_CURVE('',#2475,#2581,#1465,.T.);
#3182=EDGE_CURVE('',#2582,#2547,#1466,.T.);
#3183=EDGE_CURVE('',#2583,#2582,#1467,.T.);
#3184=EDGE_CURVE('',#2583,#2549,#1468,.T.);
#3185=EDGE_CURVE('',#2584,#2583,#1469,.T.);
#3186=EDGE_CURVE('',#2584,#2550,#1470,.T.);
#3187=EDGE_CURVE('',#2585,#2584,#2220,.T.);
#3188=EDGE_CURVE('',#2585,#2551,#1471,.T.);
#3189=EDGE_CURVE('',#2586,#2585,#1472,.T.);
#3190=EDGE_CURVE('',#2586,#2548,#1473,.T.);
#3191=EDGE_CURVE('',#2582,#2586,#1474,.T.);
#3192=EDGE_CURVE('',#2587,#2542,#1475,.T.);
#3193=EDGE_CURVE('',#2588,#2587,#1476,.T.);
#3194=EDGE_CURVE('',#2588,#2544,#1477,.T.);
#3195=EDGE_CURVE('',#2589,#2588,#1478,.T.);
#3196=EDGE_CURVE('',#2589,#2545,#1479,.T.);
#3197=EDGE_CURVE('',#2590,#2589,#1480,.T.);
#3198=EDGE_CURVE('',#2590,#2546,#1481,.T.);
#3199=EDGE_CURVE('',#2591,#2590,#2221,.T.);
#3200=EDGE_CURVE('',#2591,#2543,#1482,.T.);
#3201=EDGE_CURVE('',#2587,#2591,#1483,.T.);
#3931=ORIENTED_EDGE('',*,*,#3022,.F.);
#3932=ORIENTED_EDGE('',*,*,#3023,.T.);
#3933=ORIENTED_EDGE('',*,*,#3024,.T.);
#3934=ORIENTED_EDGE('',*,*,#3023,.F.);
#3935=ORIENTED_EDGE('',*,*,#3025,.F.);
#3936=ORIENTED_EDGE('',*,*,#3026,.T.);
#3937=ORIENTED_EDGE('',*,*,#3027,.T.);
#3938=ORIENTED_EDGE('',*,*,#3028,.F.);
#3939=ORIENTED_EDGE('',*,*,#3029,.F.);
#3940=ORIENTED_EDGE('',*,*,#3030,.T.);
#3941=ORIENTED_EDGE('',*,*,#3031,.T.);
#3942=ORIENTED_EDGE('',*,*,#3030,.F.);
#3943=ORIENTED_EDGE('',*,*,#3032,.T.);
#3944=ORIENTED_EDGE('',*,*,#3033,.T.);
#3945=ORIENTED_EDGE('',*,*,#3034,.F.);
#3946=ORIENTED_EDGE('',*,*,#3033,.F.);
#3947=ORIENTED_EDGE('',*,*,#3035,.T.);
#3948=ORIENTED_EDGE('',*,*,#3036,.T.);
#3949=ORIENTED_EDGE('',*,*,#3037,.F.);
#3950=ORIENTED_EDGE('',*,*,#3036,.F.);
#3951=ORIENTED_EDGE('',*,*,#3022,.T.);
#3952=ORIENTED_EDGE('',*,*,#3034,.T.);
#3953=ORIENTED_EDGE('',*,*,#3029,.T.);
#3954=ORIENTED_EDGE('',*,*,#3032,.F.);
#3955=ORIENTED_EDGE('',*,*,#3038,.T.);
#3956=ORIENTED_EDGE('',*,*,#3039,.T.);
#3957=ORIENTED_EDGE('',*,*,#3040,.T.);
#3958=ORIENTED_EDGE('',*,*,#3041,.T.);
#3959=ORIENTED_EDGE('',*,*,#3042,.T.);
#3960=ORIENTED_EDGE('',*,*,#3043,.T.);
#3961=ORIENTED_EDGE('',*,*,#3044,.T.);
#3962=ORIENTED_EDGE('',*,*,#3045,.T.);
#3963=ORIENTED_EDGE('',*,*,#3046,.T.);
#3964=ORIENTED_EDGE('',*,*,#3047,.T.);
#3965=ORIENTED_EDGE('',*,*,#3048,.T.);
#3966=ORIENTED_EDGE('',*,*,#3049,.T.);
#3967=ORIENTED_EDGE('',*,*,#3050,.T.);
#3968=ORIENTED_EDGE('',*,*,#3051,.T.);
#3969=ORIENTED_EDGE('',*,*,#3052,.T.);
#3970=ORIENTED_EDGE('',*,*,#3053,.T.);
#3971=ORIENTED_EDGE('',*,*,#3054,.T.);
#3972=ORIENTED_EDGE('',*,*,#3055,.T.);
#3973=ORIENTED_EDGE('',*,*,#3056,.T.);
#3974=ORIENTED_EDGE('',*,*,#3057,.T.);
#3975=ORIENTED_EDGE('',*,*,#3058,.F.);
#3976=ORIENTED_EDGE('',*,*,#3059,.F.);
#3977=ORIENTED_EDGE('',*,*,#3060,.F.);
#3978=ORIENTED_EDGE('',*,*,#3061,.F.);
#3979=ORIENTED_EDGE('',*,*,#3062,.F.);
#3980=ORIENTED_EDGE('',*,*,#3063,.F.);
#3981=ORIENTED_EDGE('',*,*,#3064,.F.);
#3982=ORIENTED_EDGE('',*,*,#3065,.F.);
#3983=ORIENTED_EDGE('',*,*,#3066,.F.);
#3984=ORIENTED_EDGE('',*,*,#3067,.F.);
#3985=ORIENTED_EDGE('',*,*,#3068,.F.);
#3986=ORIENTED_EDGE('',*,*,#3069,.F.);
#3987=ORIENTED_EDGE('',*,*,#3070,.F.);
#3988=ORIENTED_EDGE('',*,*,#3071,.F.);
#3989=ORIENTED_EDGE('',*,*,#3072,.F.);
#3990=ORIENTED_EDGE('',*,*,#3073,.F.);
#3991=ORIENTED_EDGE('',*,*,#3074,.F.);
#3992=ORIENTED_EDGE('',*,*,#3075,.F.);
#3993=ORIENTED_EDGE('',*,*,#3035,.F.);
#3994=ORIENTED_EDGE('',*,*,#3076,.F.);
#3995=ORIENTED_EDGE('',*,*,#3077,.F.);
#3996=ORIENTED_EDGE('',*,*,#3078,.F.);
#3997=ORIENTED_EDGE('',*,*,#3079,.F.);
#3998=ORIENTED_EDGE('',*,*,#3080,.F.);
#3999=ORIENTED_EDGE('',*,*,#3081,.F.);
#4000=ORIENTED_EDGE('',*,*,#3082,.F.);
#4001=ORIENTED_EDGE('',*,*,#3083,.F.);
#4002=ORIENTED_EDGE('',*,*,#3084,.F.);
#4003=ORIENTED_EDGE('',*,*,#3085,.F.);
#4004=ORIENTED_EDGE('',*,*,#3086,.F.);
#4005=ORIENTED_EDGE('',*,*,#3087,.F.);
#4006=ORIENTED_EDGE('',*,*,#3088,.F.);
#4007=ORIENTED_EDGE('',*,*,#3089,.F.);
#4008=ORIENTED_EDGE('',*,*,#3090,.F.);
#4009=ORIENTED_EDGE('',*,*,#3091,.F.);
#4010=ORIENTED_EDGE('',*,*,#3092,.F.);
#4011=ORIENTED_EDGE('',*,*,#3093,.F.);
#4012=ORIENTED_EDGE('',*,*,#3094,.F.);
#4013=ORIENTED_EDGE('',*,*,#3095,.F.);
#4014=ORIENTED_EDGE('',*,*,#3096,.F.);
#4015=ORIENTED_EDGE('',*,*,#3097,.F.);
#4016=ORIENTED_EDGE('',*,*,#3098,.F.);
#4017=ORIENTED_EDGE('',*,*,#3099,.F.);
#4018=ORIENTED_EDGE('',*,*,#3100,.F.);
#4019=ORIENTED_EDGE('',*,*,#3101,.F.);
#4020=ORIENTED_EDGE('',*,*,#3102,.F.);
#4021=ORIENTED_EDGE('',*,*,#3103,.F.);
#4022=ORIENTED_EDGE('',*,*,#3104,.F.);
#4023=ORIENTED_EDGE('',*,*,#3105,.F.);
#4024=ORIENTED_EDGE('',*,*,#3027,.F.);
#4025=ORIENTED_EDGE('',*,*,#3106,.F.);
#4026=ORIENTED_EDGE('',*,*,#3107,.F.);
#4027=ORIENTED_EDGE('',*,*,#3108,.F.);
#4028=ORIENTED_EDGE('',*,*,#3109,.F.);
#4029=ORIENTED_EDGE('',*,*,#3110,.F.);
#4030=ORIENTED_EDGE('',*,*,#3111,.F.);
#4031=ORIENTED_EDGE('',*,*,#3112,.F.);
#4032=ORIENTED_EDGE('',*,*,#3037,.T.);
#4033=ORIENTED_EDGE('',*,*,#3076,.T.);
#4034=ORIENTED_EDGE('',*,*,#3113,.F.);
#4035=ORIENTED_EDGE('',*,*,#3038,.F.);
#4036=ORIENTED_EDGE('',*,*,#3114,.T.);
#4037=ORIENTED_EDGE('',*,*,#3095,.T.);
#4038=ORIENTED_EDGE('',*,*,#3115,.F.);
#4039=ORIENTED_EDGE('',*,*,#3039,.F.);
#4040=ORIENTED_EDGE('',*,*,#3113,.T.);
#4041=ORIENTED_EDGE('',*,*,#3094,.T.);
#4042=ORIENTED_EDGE('',*,*,#3116,.F.);
#4043=ORIENTED_EDGE('',*,*,#3040,.F.);
#4044=ORIENTED_EDGE('',*,*,#3115,.T.);
#4045=ORIENTED_EDGE('',*,*,#3093,.T.);
#4046=ORIENTED_EDGE('',*,*,#3117,.F.);
#4047=ORIENTED_EDGE('',*,*,#3041,.F.);
#4048=ORIENTED_EDGE('',*,*,#3116,.T.);
#4049=ORIENTED_EDGE('',*,*,#3092,.T.);
#4050=ORIENTED_EDGE('',*,*,#3118,.F.);
#4051=ORIENTED_EDGE('',*,*,#3042,.F.);
#4052=ORIENTED_EDGE('',*,*,#3117,.T.);
#4053=ORIENTED_EDGE('',*,*,#3091,.T.);
#4054=ORIENTED_EDGE('',*,*,#3119,.F.);
#4055=ORIENTED_EDGE('',*,*,#3043,.F.);
#4056=ORIENTED_EDGE('',*,*,#3118,.T.);
#4057=ORIENTED_EDGE('',*,*,#3090,.T.);
#4058=ORIENTED_EDGE('',*,*,#3120,.F.);
#4059=ORIENTED_EDGE('',*,*,#3044,.F.);
#4060=ORIENTED_EDGE('',*,*,#3119,.T.);
#4061=ORIENTED_EDGE('',*,*,#3089,.T.);
#4062=ORIENTED_EDGE('',*,*,#3121,.F.);
#4063=ORIENTED_EDGE('',*,*,#3045,.F.);
#4064=ORIENTED_EDGE('',*,*,#3120,.T.);
#4065=ORIENTED_EDGE('',*,*,#3088,.T.);
#4066=ORIENTED_EDGE('',*,*,#3122,.F.);
#4067=ORIENTED_EDGE('',*,*,#3046,.F.);
#4068=ORIENTED_EDGE('',*,*,#3121,.T.);
#4069=ORIENTED_EDGE('',*,*,#3087,.T.);
#4070=ORIENTED_EDGE('',*,*,#3123,.F.);
#4071=ORIENTED_EDGE('',*,*,#3047,.F.);
#4072=ORIENTED_EDGE('',*,*,#3122,.T.);
#4073=ORIENTED_EDGE('',*,*,#3086,.T.);
#4074=ORIENTED_EDGE('',*,*,#3124,.F.);
#4075=ORIENTED_EDGE('',*,*,#3048,.F.);
#4076=ORIENTED_EDGE('',*,*,#3123,.T.);
#4077=ORIENTED_EDGE('',*,*,#3085,.T.);
#4078=ORIENTED_EDGE('',*,*,#3125,.F.);
#4079=ORIENTED_EDGE('',*,*,#3049,.F.);
#4080=ORIENTED_EDGE('',*,*,#3124,.T.);
#4081=ORIENTED_EDGE('',*,*,#3084,.T.);
#4082=ORIENTED_EDGE('',*,*,#3126,.F.);
#4083=ORIENTED_EDGE('',*,*,#3050,.F.);
#4084=ORIENTED_EDGE('',*,*,#3125,.T.);
#4085=ORIENTED_EDGE('',*,*,#3083,.T.);
#4086=ORIENTED_EDGE('',*,*,#3127,.F.);
#4087=ORIENTED_EDGE('',*,*,#3051,.F.);
#4088=ORIENTED_EDGE('',*,*,#3126,.T.);
#4089=ORIENTED_EDGE('',*,*,#3082,.T.);
#4090=ORIENTED_EDGE('',*,*,#3128,.F.);
#4091=ORIENTED_EDGE('',*,*,#3052,.F.);
#4092=ORIENTED_EDGE('',*,*,#3127,.T.);
#4093=ORIENTED_EDGE('',*,*,#3081,.T.);
#4094=ORIENTED_EDGE('',*,*,#3129,.F.);
#4095=ORIENTED_EDGE('',*,*,#3053,.F.);
#4096=ORIENTED_EDGE('',*,*,#3128,.T.);
#4097=ORIENTED_EDGE('',*,*,#3080,.T.);
#4098=ORIENTED_EDGE('',*,*,#3130,.F.);
#4099=ORIENTED_EDGE('',*,*,#3054,.F.);
#4100=ORIENTED_EDGE('',*,*,#3129,.T.);
#4101=ORIENTED_EDGE('',*,*,#3079,.T.);
#4102=ORIENTED_EDGE('',*,*,#3131,.F.);
#4103=ORIENTED_EDGE('',*,*,#3055,.F.);
#4104=ORIENTED_EDGE('',*,*,#3130,.T.);
#4105=ORIENTED_EDGE('',*,*,#3078,.T.);
#4106=ORIENTED_EDGE('',*,*,#3132,.F.);
#4107=ORIENTED_EDGE('',*,*,#3056,.F.);
#4108=ORIENTED_EDGE('',*,*,#3131,.T.);
#4109=ORIENTED_EDGE('',*,*,#3077,.T.);
#4110=ORIENTED_EDGE('',*,*,#3114,.F.);
#4111=ORIENTED_EDGE('',*,*,#3057,.F.);
#4112=ORIENTED_EDGE('',*,*,#3132,.T.);
#4113=ORIENTED_EDGE('',*,*,#3071,.T.);
#4114=ORIENTED_EDGE('',*,*,#3133,.F.);
#4115=ORIENTED_EDGE('',*,*,#3134,.F.);
#4116=ORIENTED_EDGE('',*,*,#3135,.T.);
#4117=ORIENTED_EDGE('',*,*,#3072,.T.);
#4118=ORIENTED_EDGE('',*,*,#3135,.F.);
#4119=ORIENTED_EDGE('',*,*,#3136,.F.);
#4120=ORIENTED_EDGE('',*,*,#3137,.T.);
#4121=ORIENTED_EDGE('',*,*,#3073,.T.);
#4122=ORIENTED_EDGE('',*,*,#3137,.F.);
#4123=ORIENTED_EDGE('',*,*,#3138,.F.);
#4124=ORIENTED_EDGE('',*,*,#3139,.T.);
#4125=ORIENTED_EDGE('',*,*,#3074,.T.);
#4126=ORIENTED_EDGE('',*,*,#3139,.F.);
#4127=ORIENTED_EDGE('',*,*,#3140,.F.);
#4128=ORIENTED_EDGE('',*,*,#3141,.T.);
#4129=ORIENTED_EDGE('',*,*,#3075,.T.);
#4130=ORIENTED_EDGE('',*,*,#3141,.F.);
#4131=ORIENTED_EDGE('',*,*,#3142,.F.);
#4132=ORIENTED_EDGE('',*,*,#3133,.T.);
#4133=ORIENTED_EDGE('',*,*,#3134,.T.);
#4134=ORIENTED_EDGE('',*,*,#3142,.T.);
#4135=ORIENTED_EDGE('',*,*,#3140,.T.);
#4136=ORIENTED_EDGE('',*,*,#3138,.T.);
#4137=ORIENTED_EDGE('',*,*,#3136,.T.);
#4138=ORIENTED_EDGE('',*,*,#3066,.T.);
#4139=ORIENTED_EDGE('',*,*,#3143,.F.);
#4140=ORIENTED_EDGE('',*,*,#3144,.F.);
#4141=ORIENTED_EDGE('',*,*,#3145,.T.);
#4142=ORIENTED_EDGE('',*,*,#3067,.T.);
#4143=ORIENTED_EDGE('',*,*,#3145,.F.);
#4144=ORIENTED_EDGE('',*,*,#3146,.F.);
#4145=ORIENTED_EDGE('',*,*,#3147,.T.);
#4146=ORIENTED_EDGE('',*,*,#3068,.T.);
#4147=ORIENTED_EDGE('',*,*,#3147,.F.);
#4148=ORIENTED_EDGE('',*,*,#3148,.F.);
#4149=ORIENTED_EDGE('',*,*,#3149,.T.);
#4150=ORIENTED_EDGE('',*,*,#3069,.T.);
#4151=ORIENTED_EDGE('',*,*,#3149,.F.);
#4152=ORIENTED_EDGE('',*,*,#3150,.F.);
#4153=ORIENTED_EDGE('',*,*,#3151,.T.);
#4154=ORIENTED_EDGE('',*,*,#3070,.T.);
#4155=ORIENTED_EDGE('',*,*,#3151,.F.);
#4156=ORIENTED_EDGE('',*,*,#3152,.F.);
#4157=ORIENTED_EDGE('',*,*,#3143,.T.);
#4158=ORIENTED_EDGE('',*,*,#3144,.T.);
#4159=ORIENTED_EDGE('',*,*,#3152,.T.);
#4160=ORIENTED_EDGE('',*,*,#3150,.T.);
#4161=ORIENTED_EDGE('',*,*,#3148,.T.);
#4162=ORIENTED_EDGE('',*,*,#3146,.T.);
#4163=ORIENTED_EDGE('',*,*,#3058,.T.);
#4164=ORIENTED_EDGE('',*,*,#3153,.F.);
#4165=ORIENTED_EDGE('',*,*,#3154,.F.);
#4166=ORIENTED_EDGE('',*,*,#3155,.T.);
#4167=ORIENTED_EDGE('',*,*,#3059,.T.);
#4168=ORIENTED_EDGE('',*,*,#3155,.F.);
#4169=ORIENTED_EDGE('',*,*,#3156,.F.);
#4170=ORIENTED_EDGE('',*,*,#3157,.T.);
#4171=ORIENTED_EDGE('',*,*,#3060,.T.);
#4172=ORIENTED_EDGE('',*,*,#3157,.F.);
#4173=ORIENTED_EDGE('',*,*,#3158,.F.);
#4174=ORIENTED_EDGE('',*,*,#3159,.T.);
#4175=ORIENTED_EDGE('',*,*,#3061,.T.);
#4176=ORIENTED_EDGE('',*,*,#3159,.F.);
#4177=ORIENTED_EDGE('',*,*,#3160,.F.);
#4178=ORIENTED_EDGE('',*,*,#3161,.T.);
#4179=ORIENTED_EDGE('',*,*,#3062,.T.);
#4180=ORIENTED_EDGE('',*,*,#3161,.F.);
#4181=ORIENTED_EDGE('',*,*,#3162,.F.);
#4182=ORIENTED_EDGE('',*,*,#3163,.T.);
#4183=ORIENTED_EDGE('',*,*,#3063,.T.);
#4184=ORIENTED_EDGE('',*,*,#3163,.F.);
#4185=ORIENTED_EDGE('',*,*,#3164,.F.);
#4186=ORIENTED_EDGE('',*,*,#3165,.T.);
#4187=ORIENTED_EDGE('',*,*,#3064,.T.);
#4188=ORIENTED_EDGE('',*,*,#3165,.F.);
#4189=ORIENTED_EDGE('',*,*,#3166,.F.);
#4190=ORIENTED_EDGE('',*,*,#3167,.T.);
#4191=ORIENTED_EDGE('',*,*,#3065,.T.);
#4192=ORIENTED_EDGE('',*,*,#3167,.F.);
#4193=ORIENTED_EDGE('',*,*,#3168,.F.);
#4194=ORIENTED_EDGE('',*,*,#3153,.T.);
#4195=ORIENTED_EDGE('',*,*,#3154,.T.);
#4196=ORIENTED_EDGE('',*,*,#3168,.T.);
#4197=ORIENTED_EDGE('',*,*,#3166,.T.);
#4198=ORIENTED_EDGE('',*,*,#3164,.T.);
#4199=ORIENTED_EDGE('',*,*,#3162,.T.);
#4200=ORIENTED_EDGE('',*,*,#3160,.T.);
#4201=ORIENTED_EDGE('',*,*,#3158,.T.);
#4202=ORIENTED_EDGE('',*,*,#3156,.T.);
#4203=ORIENTED_EDGE('',*,*,#3031,.F.);
#4204=ORIENTED_EDGE('',*,*,#3106,.T.);
#4205=ORIENTED_EDGE('',*,*,#3026,.F.);
#4206=ORIENTED_EDGE('',*,*,#3169,.F.);
#4207=ORIENTED_EDGE('',*,*,#3170,.T.);
#4208=ORIENTED_EDGE('',*,*,#3107,.T.);
#4209=ORIENTED_EDGE('',*,*,#3170,.F.);
#4210=ORIENTED_EDGE('',*,*,#3171,.F.);
#4211=ORIENTED_EDGE('',*,*,#3172,.T.);
#4212=ORIENTED_EDGE('',*,*,#3108,.T.);
#4213=ORIENTED_EDGE('',*,*,#3172,.F.);
#4214=ORIENTED_EDGE('',*,*,#3173,.F.);
#4215=ORIENTED_EDGE('',*,*,#3174,.T.);
#4216=ORIENTED_EDGE('',*,*,#3109,.T.);
#4217=ORIENTED_EDGE('',*,*,#3174,.F.);
#4218=ORIENTED_EDGE('',*,*,#3175,.F.);
#4219=ORIENTED_EDGE('',*,*,#3176,.T.);
#4220=ORIENTED_EDGE('',*,*,#3110,.T.);
#4221=ORIENTED_EDGE('',*,*,#3176,.F.);
#4222=ORIENTED_EDGE('',*,*,#3177,.F.);
#4223=ORIENTED_EDGE('',*,*,#3178,.T.);
#4224=ORIENTED_EDGE('',*,*,#3111,.T.);
#4225=ORIENTED_EDGE('',*,*,#3178,.F.);
#4226=ORIENTED_EDGE('',*,*,#3179,.F.);
#4227=ORIENTED_EDGE('',*,*,#3180,.T.);
#4228=ORIENTED_EDGE('',*,*,#3112,.T.);
#4229=ORIENTED_EDGE('',*,*,#3180,.F.);
#4230=ORIENTED_EDGE('',*,*,#3181,.F.);
#4231=ORIENTED_EDGE('',*,*,#3028,.T.);
#4232=ORIENTED_EDGE('',*,*,#3169,.T.);
#4233=ORIENTED_EDGE('',*,*,#3025,.T.);
#4234=ORIENTED_EDGE('',*,*,#3181,.T.);
#4235=ORIENTED_EDGE('',*,*,#3179,.T.);
#4236=ORIENTED_EDGE('',*,*,#3177,.T.);
#4237=ORIENTED_EDGE('',*,*,#3175,.T.);
#4238=ORIENTED_EDGE('',*,*,#3173,.T.);
#4239=ORIENTED_EDGE('',*,*,#3171,.T.);
#4240=ORIENTED_EDGE('',*,*,#3024,.F.);
#4241=ORIENTED_EDGE('',*,*,#3102,.T.);
#4242=ORIENTED_EDGE('',*,*,#3182,.F.);
#4243=ORIENTED_EDGE('',*,*,#3183,.F.);
#4244=ORIENTED_EDGE('',*,*,#3184,.T.);
#4245=ORIENTED_EDGE('',*,*,#3103,.T.);
#4246=ORIENTED_EDGE('',*,*,#3184,.F.);
#4247=ORIENTED_EDGE('',*,*,#3185,.F.);
#4248=ORIENTED_EDGE('',*,*,#3186,.T.);
#4249=ORIENTED_EDGE('',*,*,#3104,.T.);
#4250=ORIENTED_EDGE('',*,*,#3186,.F.);
#4251=ORIENTED_EDGE('',*,*,#3187,.F.);
#4252=ORIENTED_EDGE('',*,*,#3188,.T.);
#4253=ORIENTED_EDGE('',*,*,#3105,.T.);
#4254=ORIENTED_EDGE('',*,*,#3188,.F.);
#4255=ORIENTED_EDGE('',*,*,#3189,.F.);
#4256=ORIENTED_EDGE('',*,*,#3190,.T.);
#4257=ORIENTED_EDGE('',*,*,#3101,.T.);
#4258=ORIENTED_EDGE('',*,*,#3190,.F.);
#4259=ORIENTED_EDGE('',*,*,#3191,.F.);
#4260=ORIENTED_EDGE('',*,*,#3182,.T.);
#4261=ORIENTED_EDGE('',*,*,#3183,.T.);
#4262=ORIENTED_EDGE('',*,*,#3191,.T.);
#4263=ORIENTED_EDGE('',*,*,#3189,.T.);
#4264=ORIENTED_EDGE('',*,*,#3187,.T.);
#4265=ORIENTED_EDGE('',*,*,#3185,.T.);
#4266=ORIENTED_EDGE('',*,*,#3097,.T.);
#4267=ORIENTED_EDGE('',*,*,#3192,.F.);
#4268=ORIENTED_EDGE('',*,*,#3193,.F.);
#4269=ORIENTED_EDGE('',*,*,#3194,.T.);
#4270=ORIENTED_EDGE('',*,*,#3098,.T.);
#4271=ORIENTED_EDGE('',*,*,#3194,.F.);
#4272=ORIENTED_EDGE('',*,*,#3195,.F.);
#4273=ORIENTED_EDGE('',*,*,#3196,.T.);
#4274=ORIENTED_EDGE('',*,*,#3099,.T.);
#4275=ORIENTED_EDGE('',*,*,#3196,.F.);
#4276=ORIENTED_EDGE('',*,*,#3197,.F.);
#4277=ORIENTED_EDGE('',*,*,#3198,.T.);
#4278=ORIENTED_EDGE('',*,*,#3100,.T.);
#4279=ORIENTED_EDGE('',*,*,#3198,.F.);
#4280=ORIENTED_EDGE('',*,*,#3199,.F.);
#4281=ORIENTED_EDGE('',*,*,#3200,.T.);
#4282=ORIENTED_EDGE('',*,*,#3096,.T.);
#4283=ORIENTED_EDGE('',*,*,#3200,.F.);
#4284=ORIENTED_EDGE('',*,*,#3201,.F.);
#4285=ORIENTED_EDGE('',*,*,#3192,.T.);
#4286=ORIENTED_EDGE('',*,*,#3193,.T.);
#4287=ORIENTED_EDGE('',*,*,#3201,.T.);
#4288=ORIENTED_EDGE('',*,*,#3199,.T.);
#4289=ORIENTED_EDGE('',*,*,#3197,.T.);
#4290=ORIENTED_EDGE('',*,*,#3195,.T.);
#5195=CYLINDRICAL_SURFACE('',#5784,3.5);
#5196=CYLINDRICAL_SURFACE('',#5787,4.5);
#5197=CYLINDRICAL_SURFACE('',#5790,3.5);
#5198=CYLINDRICAL_SURFACE('',#5793,2.5);
#5199=CYLINDRICAL_SURFACE('',#5796,2.5);
#5200=CYLINDRICAL_SURFACE('',#5818,6.50000000000001);
#5201=CYLINDRICAL_SURFACE('',#5820,10.);
#5202=CYLINDRICAL_SURFACE('',#5827,23.);
#5203=CYLINDRICAL_SURFACE('',#5840,24.9999999999999);
#5204=CYLINDRICAL_SURFACE('',#5846,24.9999999999999);
#5205=CYLINDRICAL_SURFACE('',#5850,4.5);
#5206=CYLINDRICAL_SURFACE('',#5856,12.);
#5207=CYLINDRICAL_SURFACE('',#5863,12.);
#5208=CYLINDRICAL_SURFACE('',#5872,24.9999999999999);
#5209=CYLINDRICAL_SURFACE('',#5880,24.9999999999999);
#5325=ADVANCED_FACE('',(#608),#5195,.T.);
#5326=ADVANCED_FACE('',(#609),#5196,.T.);
#5327=ADVANCED_FACE('',(#610),#5197,.T.);
#5328=ADVANCED_FACE('',(#611),#5198,.F.);
#5329=ADVANCED_FACE('',(#612),#5199,.F.);
#5330=ADVANCED_FACE('',(#613,#355),#425,.F.);
#5331=ADVANCED_FACE('',(#614,#356),#426,.T.);
#5332=ADVANCED_FACE('',(#615,#357,#358,#359,#360),#427,.T.);
#5333=ADVANCED_FACE('',(#616,#361,#362,#363,#364),#428,.F.);
#5334=ADVANCED_FACE('',(#617),#429,.F.);
#5335=ADVANCED_FACE('',(#618),#430,.F.);
#5336=ADVANCED_FACE('',(#619),#5200,.T.);
#5337=ADVANCED_FACE('',(#620),#431,.F.);
#5338=ADVANCED_FACE('',(#621),#5201,.F.);
#5339=ADVANCED_FACE('',(#622),#432,.F.);
#5340=ADVANCED_FACE('',(#623),#433,.F.);
#5341=ADVANCED_FACE('',(#624),#434,.F.);
#5342=ADVANCED_FACE('',(#625),#435,.F.);
#5343=ADVANCED_FACE('',(#626),#436,.F.);
#5344=ADVANCED_FACE('',(#627),#437,.F.);
#5345=ADVANCED_FACE('',(#628),#5202,.F.);
#5346=ADVANCED_FACE('',(#629),#438,.F.);
#5347=ADVANCED_FACE('',(#630),#439,.F.);
#5348=ADVANCED_FACE('',(#631),#440,.F.);
#5349=ADVANCED_FACE('',(#632),#441,.F.);
#5350=ADVANCED_FACE('',(#633),#442,.F.);
#5351=ADVANCED_FACE('',(#634),#443,.F.);
#5352=ADVANCED_FACE('',(#635),#444,.F.);
#5353=ADVANCED_FACE('',(#636),#445,.F.);
#5354=ADVANCED_FACE('',(#637),#446,.F.);
#5355=ADVANCED_FACE('',(#638),#447,.F.);
#5356=ADVANCED_FACE('',(#639),#448,.F.);
#5357=ADVANCED_FACE('',(#640),#449,.F.);
#5358=ADVANCED_FACE('',(#641),#5203,.T.);
#5359=ADVANCED_FACE('',(#642),#450,.T.);
#5360=ADVANCED_FACE('',(#643),#451,.F.);
#5361=ADVANCED_FACE('',(#644),#452,.F.);
#5362=ADVANCED_FACE('',(#645),#453,.F.);
#5363=ADVANCED_FACE('',(#646),#5204,.T.);
#5364=ADVANCED_FACE('',(#647),#454,.F.);
#5365=ADVANCED_FACE('',(#648),#455,.T.);
#5366=ADVANCED_FACE('',(#649),#5205,.T.);
#5367=ADVANCED_FACE('',(#650),#456,.F.);
#5368=ADVANCED_FACE('',(#651),#457,.F.);
#5369=ADVANCED_FACE('',(#652),#458,.F.);
#5370=ADVANCED_FACE('',(#653),#459,.F.);
#5371=ADVANCED_FACE('',(#654),#5206,.T.);
#5372=ADVANCED_FACE('',(#655),#460,.F.);
#5373=ADVANCED_FACE('',(#656),#461,.F.);
#5374=ADVANCED_FACE('',(#657,#365),#462,.T.);
#5375=ADVANCED_FACE('',(#658),#463,.F.);
#5376=ADVANCED_FACE('',(#659),#464,.F.);
#5377=ADVANCED_FACE('',(#660),#5207,.T.);
#5378=ADVANCED_FACE('',(#661),#465,.F.);
#5379=ADVANCED_FACE('',(#662),#466,.F.);
#5380=ADVANCED_FACE('',(#663),#467,.F.);
#5381=ADVANCED_FACE('',(#664),#468,.F.);
#5382=ADVANCED_FACE('',(#665,#366),#469,.T.);
#5383=ADVANCED_FACE('',(#666),#470,.F.);
#5384=ADVANCED_FACE('',(#667),#471,.F.);
#5385=ADVANCED_FACE('',(#668),#5208,.T.);
#5386=ADVANCED_FACE('',(#669),#472,.F.);
#5387=ADVANCED_FACE('',(#670),#473,.F.);
#5388=ADVANCED_FACE('',(#671),#474,.T.);
#5389=ADVANCED_FACE('',(#672),#475,.F.);
#5390=ADVANCED_FACE('',(#673),#476,.F.);
#5391=ADVANCED_FACE('',(#674),#477,.F.);
#5392=ADVANCED_FACE('',(#675),#5209,.T.);
#5393=ADVANCED_FACE('',(#676),#478,.F.);
#5394=ADVANCED_FACE('',(#677),#479,.T.);
#5583=CLOSED_SHELL('',(#5325,#5326,#5327,#5328,#5329,#5330,#5331,#5332,
#5333,#5334,#5335,#5336,#5337,#5338,#5339,#5340,#5341,#5342,#5343,#5344,
#5345,#5346,#5347,#5348,#5349,#5350,#5351,#5352,#5353,#5354,#5355,#5356,
#5357,#5358,#5359,#5360,#5361,#5362,#5363,#5364,#5365,#5366,#5367,#5368,
#5369,#5370,#5371,#5372,#5373,#5374,#5375,#5376,#5377,#5378,#5379,#5380,
#5381,#5382,#5383,#5384,#5385,#5386,#5387,#5388,#5389,#5390,#5391,#5392,
#5393,#5394));
#5783=AXIS2_PLACEMENT_3D('',#8065,#6530,#6531);
#5784=AXIS2_PLACEMENT_3D('',#8066,#6532,#6533);
#5785=AXIS2_PLACEMENT_3D('',#8068,#6534,#6535);
#5786=AXIS2_PLACEMENT_3D('',#8071,#6537,#6538);
#5787=AXIS2_PLACEMENT_3D('',#8072,#6539,#6540);
#5788=AXIS2_PLACEMENT_3D('',#8075,#6541,#6542);
#5789=AXIS2_PLACEMENT_3D('',#8079,#6544,#6545);
#5790=AXIS2_PLACEMENT_3D('',#8081,#6547,#6548);
#5791=AXIS2_PLACEMENT_3D('',#8083,#6549,#6550);
#5792=AXIS2_PLACEMENT_3D('',#8086,#6552,#6553);
#5793=AXIS2_PLACEMENT_3D('',#8087,#6554,#6555);
#5794=AXIS2_PLACEMENT_3D('',#8089,#6556,#6557);
#5795=AXIS2_PLACEMENT_3D('',#8092,#6559,#6560);
#5796=AXIS2_PLACEMENT_3D('',#8093,#6561,#6562);
#5797=AXIS2_PLACEMENT_3D('',#8095,#6563,#6564);
#5798=AXIS2_PLACEMENT_3D('',#8098,#6566,#6567);
#5799=AXIS2_PLACEMENT_3D('',#8099,#6568,#6569);
#5800=AXIS2_PLACEMENT_3D('',#8100,#6570,#6571);
#5801=AXIS2_PLACEMENT_3D('',#8101,#6572,#6573);
#5802=AXIS2_PLACEMENT_3D('',#8108,#6576,#6577);
#5803=AXIS2_PLACEMENT_3D('',#8112,#6579,#6580);
#5804=AXIS2_PLACEMENT_3D('',#8126,#6587,#6588);
#5805=AXIS2_PLACEMENT_3D('',#8144,#6597,#6598);
#5806=AXIS2_PLACEMENT_3D('',#8154,#6603,#6604);
#5807=AXIS2_PLACEMENT_3D('',#8166,#6610,#6611);
#5808=AXIS2_PLACEMENT_3D('',#8177,#6617,#6618);
#5809=AXIS2_PLACEMENT_3D('',#8178,#6619,#6620);
#5810=AXIS2_PLACEMENT_3D('',#8199,#6630,#6631);
#5811=AXIS2_PLACEMENT_3D('',#8213,#6638,#6639);
#5812=AXIS2_PLACEMENT_3D('',#8217,#6641,#6642);
#5813=AXIS2_PLACEMENT_3D('',#8228,#6648,#6649);
#5814=AXIS2_PLACEMENT_3D('',#8237,#6653,#6654);
#5815=AXIS2_PLACEMENT_3D('',#8244,#6658,#6659);
#5816=AXIS2_PLACEMENT_3D('',#8252,#6664,#6665);
#5817=AXIS2_PLACEMENT_3D('',#8255,#6668,#6669);
#5818=AXIS2_PLACEMENT_3D('',#8257,#6671,#6672);
#5819=AXIS2_PLACEMENT_3D('',#8259,#6674,#6675);
#5820=AXIS2_PLACEMENT_3D('',#8261,#6677,#6678);
#5821=AXIS2_PLACEMENT_3D('',#8263,#6680,#6681);
#5822=AXIS2_PLACEMENT_3D('',#8265,#6683,#6684);
#5823=AXIS2_PLACEMENT_3D('',#8267,#6686,#6687);
#5824=AXIS2_PLACEMENT_3D('',#8269,#6689,#6690);
#5825=AXIS2_PLACEMENT_3D('',#8271,#6692,#6693);
#5826=AXIS2_PLACEMENT_3D('',#8273,#6695,#6696);
#5827=AXIS2_PLACEMENT_3D('',#8275,#6698,#6699);
#5828=AXIS2_PLACEMENT_3D('',#8277,#6701,#6702);
#5829=AXIS2_PLACEMENT_3D('',#8279,#6704,#6705);
#5830=AXIS2_PLACEMENT_3D('',#8281,#6707,#6708);
#5831=AXIS2_PLACEMENT_3D('',#8283,#6710,#6711);
#5832=AXIS2_PLACEMENT_3D('',#8285,#6713,#6714);
#5833=AXIS2_PLACEMENT_3D('',#8287,#6716,#6717);
#5834=AXIS2_PLACEMENT_3D('',#8289,#6719,#6720);
#5835=AXIS2_PLACEMENT_3D('',#8291,#6722,#6723);
#5836=AXIS2_PLACEMENT_3D('',#8292,#6724,#6725);
#5837=AXIS2_PLACEMENT_3D('',#8298,#6729,#6730);
#5838=AXIS2_PLACEMENT_3D('',#8302,#6733,#6734);
#5839=AXIS2_PLACEMENT_3D('',#8306,#6737,#6738);
#5840=AXIS2_PLACEMENT_3D('',#8310,#6741,#6742);
#5841=AXIS2_PLACEMENT_3D('',#8311,#6743,#6744);
#5842=AXIS2_PLACEMENT_3D('',#8312,#6745,#6746);
#5843=AXIS2_PLACEMENT_3D('',#8313,#6747,#6748);
#5844=AXIS2_PLACEMENT_3D('',#8319,#6752,#6753);
#5845=AXIS2_PLACEMENT_3D('',#8323,#6756,#6757);
#5846=AXIS2_PLACEMENT_3D('',#8327,#6760,#6761);
#5847=AXIS2_PLACEMENT_3D('',#8329,#6762,#6763);
#5848=AXIS2_PLACEMENT_3D('',#8331,#6765,#6766);
#5849=AXIS2_PLACEMENT_3D('',#8333,#6768,#6769);
#5850=AXIS2_PLACEMENT_3D('',#8334,#6770,#6771);
#5851=AXIS2_PLACEMENT_3D('',#8338,#6773,#6774);
#5852=AXIS2_PLACEMENT_3D('',#8340,#6776,#6777);
#5853=AXIS2_PLACEMENT_3D('',#8344,#6780,#6781);
#5854=AXIS2_PLACEMENT_3D('',#8348,#6784,#6785);
#5855=AXIS2_PLACEMENT_3D('',#8352,#6788,#6789);
#5856=AXIS2_PLACEMENT_3D('',#8356,#6792,#6793);
#5857=AXIS2_PLACEMENT_3D('',#8358,#6794,#6795);
#5858=AXIS2_PLACEMENT_3D('',#8360,#6797,#6798);
#5859=AXIS2_PLACEMENT_3D('',#8364,#6801,#6802);
#5860=AXIS2_PLACEMENT_3D('',#8366,#6804,#6805);
#5861=AXIS2_PLACEMENT_3D('',#8367,#6806,#6807);
#5862=AXIS2_PLACEMENT_3D('',#8371,#6810,#6811);
#5863=AXIS2_PLACEMENT_3D('',#8375,#6814,#6815);
#5864=AXIS2_PLACEMENT_3D('',#8377,#6816,#6817);
#5865=AXIS2_PLACEMENT_3D('',#8379,#6819,#6820);
#5866=AXIS2_PLACEMENT_3D('',#8383,#6823,#6824);
#5867=AXIS2_PLACEMENT_3D('',#8387,#6827,#6828);
#5868=AXIS2_PLACEMENT_3D('',#8391,#6831,#6832);
#5869=AXIS2_PLACEMENT_3D('',#8393,#6834,#6835);
#5870=AXIS2_PLACEMENT_3D('',#8394,#6836,#6837);
#5871=AXIS2_PLACEMENT_3D('',#8400,#6841,#6842);
#5872=AXIS2_PLACEMENT_3D('',#8404,#6845,#6846);
#5873=AXIS2_PLACEMENT_3D('',#8406,#6847,#6848);
#5874=AXIS2_PLACEMENT_3D('',#8408,#6850,#6851);
#5875=AXIS2_PLACEMENT_3D('',#8412,#6854,#6855);
#5876=AXIS2_PLACEMENT_3D('',#8414,#6857,#6858);
#5877=AXIS2_PLACEMENT_3D('',#8415,#6859,#6860);
#5878=AXIS2_PLACEMENT_3D('',#8421,#6864,#6865);
#5879=AXIS2_PLACEMENT_3D('',#8425,#6868,#6869);
#5880=AXIS2_PLACEMENT_3D('',#8429,#6872,#6873);
#5881=AXIS2_PLACEMENT_3D('',#8431,#6874,#6875);
#5882=AXIS2_PLACEMENT_3D('',#8433,#6877,#6878);
#5883=AXIS2_PLACEMENT_3D('',#8435,#6880,#6881);
#6530=DIRECTION('axis',(0.,0.,1.));
#6531=DIRECTION('refdir',(1.,0.,0.));
#6532=DIRECTION('center_axis',(0.,-1.,0.));
#6533=DIRECTION('ref_axis',(0.,0.,-1.));
#6534=DIRECTION('center_axis',(0.,-1.,0.));
#6535=DIRECTION('ref_axis',(0.,0.,-1.));
#6536=DIRECTION('',(0.,1.,0.));
#6537=DIRECTION('center_axis',(0.,-1.,0.));
#6538=DIRECTION('ref_axis',(0.,0.,-1.));
#6539=DIRECTION('center_axis',(0.,-1.,0.));
#6540=DIRECTION('ref_axis',(0.,0.,-1.));
#6541=DIRECTION('center_axis',(0.,1.,0.));
#6542=DIRECTION('ref_axis',(0.,0.,-1.));
#6543=DIRECTION('',(0.,-1.,0.));
#6544=DIRECTION('center_axis',(0.,1.,0.));
#6545=DIRECTION('ref_axis',(0.,0.,-1.));
#6546=DIRECTION('',(0.,-1.,0.));
#6547=DIRECTION('center_axis',(0.,1.,0.));
#6548=DIRECTION('ref_axis',(0.,0.,1.));
#6549=DIRECTION('center_axis',(0.,1.,0.));
#6550=DIRECTION('ref_axis',(0.,0.,1.));
#6551=DIRECTION('',(0.,-1.,0.));
#6552=DIRECTION('center_axis',(0.,1.,0.));
#6553=DIRECTION('ref_axis',(0.,0.,1.));
#6554=DIRECTION('center_axis',(0.,-1.,0.));
#6555=DIRECTION('ref_axis',(0.,0.,-1.));
#6556=DIRECTION('center_axis',(0.,1.,0.));
#6557=DIRECTION('ref_axis',(0.,0.,1.));
#6558=DIRECTION('',(0.,-1.,0.));
#6559=DIRECTION('center_axis',(0.,1.,0.));
#6560=DIRECTION('ref_axis',(0.,0.,1.));
#6561=DIRECTION('center_axis',(0.,-1.,0.));
#6562=DIRECTION('ref_axis',(0.,0.,-1.));
#6563=DIRECTION('center_axis',(0.,1.,0.));
#6564=DIRECTION('ref_axis',(0.,0.,1.));
#6565=DIRECTION('',(0.,-1.,0.));
#6566=DIRECTION('center_axis',(0.,1.,0.));
#6567=DIRECTION('ref_axis',(0.,0.,1.));
#6568=DIRECTION('center_axis',(0.,1.,0.));
#6569=DIRECTION('ref_axis',(0.,0.,1.));
#6570=DIRECTION('center_axis',(0.,1.,0.));
#6571=DIRECTION('ref_axis',(0.,0.,1.));
#6572=DIRECTION('center_axis',(0.,1.,0.));
#6573=DIRECTION('ref_axis',(0.,0.,1.));
#6574=DIRECTION('',(-0.500000000000001,0.,0.866025403784438));
#6575=DIRECTION('',(9.91270557701033E-17,0.,1.));
#6576=DIRECTION('center_axis',(0.,1.,0.));
#6577=DIRECTION('ref_axis',(0.,0.,1.));
#6578=DIRECTION('',(0.,0.,-1.));
#6579=DIRECTION('center_axis',(0.,-1.,0.));
#6580=DIRECTION('ref_axis',(0.,0.,1.));
#6581=DIRECTION('',(1.,0.,0.));
#6582=DIRECTION('',(0.707106781186576,0.,-0.707106781186519));
#6583=DIRECTION('',(-0.707106781186549,0.,-0.707106781186546));
#6584=DIRECTION('',(0.707106781186548,0.,-0.707106781186547));
#6585=DIRECTION('',(-0.707106781186548,0.,-0.707106781186547));
#6586=DIRECTION('',(0.707106781186546,0.,-0.707106781186549));
#6587=DIRECTION('center_axis',(0.,-1.,0.));
#6588=DIRECTION('ref_axis',(0.,0.,1.));
#6589=DIRECTION('',(-0.819152044289008,0.,-0.573576436351023));
#6590=DIRECTION('',(0.573576436351062,0.,-0.819152044288981));
#6591=DIRECTION('',(-0.819152044288987,0.,-0.573576436351053));
#6592=DIRECTION('',(0.573576436351036,0.,-0.819152044288999));
#6593=DIRECTION('',(-0.819152044288996,0.,-0.57357643635104));
#6594=DIRECTION('',(0.573576436351043,0.,-0.819152044288994));
#6595=DIRECTION('',(-0.173648177666936,0.,-0.984807753012207));
#6596=DIRECTION('',(-0.984807753012208,0.,0.173648177666932));
#6597=DIRECTION('center_axis',(0.,-1.,0.));
#6598=DIRECTION('ref_axis',(0.,0.,1.));
#6599=DIRECTION('',(1.,0.,0.));
#6600=DIRECTION('',(4.45418905079446E-17,0.,1.));
#6601=DIRECTION('',(-1.,0.,0.));
#6602=DIRECTION('',(0.,0.,-1.));
#6603=DIRECTION('center_axis',(0.,-1.,0.));
#6604=DIRECTION('ref_axis',(0.,0.,1.));
#6605=DIRECTION('',(8.19364478113207E-17,0.,-1.));
#6606=DIRECTION('',(1.,0.,0.));
#6607=DIRECTION('',(1.,0.,0.));
#6608=DIRECTION('',(7.41956747162227E-17,0.,1.));
#6609=DIRECTION('',(-0.866025403784438,0.,-0.5));
#6610=DIRECTION('center_axis',(0.,-1.,0.));
#6611=DIRECTION('ref_axis',(0.,0.,1.));
#6612=DIRECTION('',(-5.78241158658935E-16,0.,-1.));
#6613=DIRECTION('',(0.866025403784439,0.,0.499999999999999));
#6614=DIRECTION('',(-0.5,0.,0.866025403784439));
#6615=DIRECTION('',(-0.984807753012207,0.,0.173648177666934));
#6616=DIRECTION('',(-0.173648177666936,0.,-0.984807753012207));
#6617=DIRECTION('center_axis',(0.,-1.,0.));
#6618=DIRECTION('ref_axis',(0.,0.,1.));
#6619=DIRECTION('center_axis',(0.,1.,0.));
#6620=DIRECTION('ref_axis',(0.,0.,1.));
#6621=DIRECTION('',(-0.500000000000001,0.,0.866025403784438));
#6622=DIRECTION('',(-0.984807753012208,0.,0.173648177666932));
#6623=DIRECTION('',(-0.173648177666936,0.,-0.984807753012207));
#6624=DIRECTION('',(0.573576436351043,0.,-0.819152044288994));
#6625=DIRECTION('',(-0.819152044288996,0.,-0.57357643635104));
#6626=DIRECTION('',(0.573576436351036,0.,-0.819152044288999));
#6627=DIRECTION('',(-0.819152044288987,0.,-0.573576436351053));
#6628=DIRECTION('',(0.573576436351062,0.,-0.819152044288981));
#6629=DIRECTION('',(-0.819152044289008,0.,-0.573576436351023));
#6630=DIRECTION('center_axis',(0.,-1.,0.));
#6631=DIRECTION('ref_axis',(0.,0.,1.));
#6632=DIRECTION('',(0.707106781186546,0.,-0.707106781186549));
#6633=DIRECTION('',(-0.707106781186548,0.,-0.707106781186547));
#6634=DIRECTION('',(0.707106781186548,0.,-0.707106781186547));
#6635=DIRECTION('',(-0.707106781186549,0.,-0.707106781186546));
#6636=DIRECTION('',(0.707106781186576,0.,-0.707106781186519));
#6637=DIRECTION('',(1.,0.,0.));
#6638=DIRECTION('center_axis',(0.,-1.,0.));
#6639=DIRECTION('ref_axis',(0.,0.,1.));
#6640=DIRECTION('',(0.,0.,-1.));
#6641=DIRECTION('center_axis',(0.,1.,0.));
#6642=DIRECTION('ref_axis',(0.,0.,1.));
#6643=DIRECTION('',(9.91270557701033E-17,0.,1.));
#6644=DIRECTION('',(0.866025403784438,0.,0.5));
#6645=DIRECTION('',(-7.41956747162227E-17,0.,-1.));
#6646=DIRECTION('',(-1.,0.,0.));
#6647=DIRECTION('',(5.20417042793039E-15,0.,1.));
#6648=DIRECTION('center_axis',(0.,1.,0.));
#6649=DIRECTION('ref_axis',(0.,0.,-1.));
#6650=DIRECTION('',(0.984807753012207,0.,-0.173648177666934));
#6651=DIRECTION('',(0.5,0.,-0.866025403784439));
#6652=DIRECTION('',(-0.866025403784439,0.,-0.499999999999999));
#6653=DIRECTION('center_axis',(0.,1.,0.));
#6654=DIRECTION('ref_axis',(0.,0.,-1.));
#6655=DIRECTION('',(0.173648177666936,0.,0.984807753012207));
#6656=DIRECTION('',(-1.,0.,-4.33680868994201E-16));
#6657=DIRECTION('',(-8.19364478113207E-17,0.,1.));
#6658=DIRECTION('center_axis',(0.,1.,0.));
#6659=DIRECTION('ref_axis',(0.,0.,-1.));
#6660=DIRECTION('',(2.89120579329468E-16,0.,1.));
#6661=DIRECTION('',(1.,0.,0.));
#6662=DIRECTION('',(-4.45418905079446E-17,0.,-1.));
#6663=DIRECTION('',(-1.,0.,0.));
#6664=DIRECTION('center_axis',(0.866025403784438,0.,0.500000000000001));
#6665=DIRECTION('ref_axis',(0.500000000000001,0.,-0.866025403784438));
#6666=DIRECTION('',(0.,-1.,0.));
#6667=DIRECTION('',(0.,-1.,0.));
#6668=DIRECTION('center_axis',(1.,0.,-9.91270557701033E-17));
#6669=DIRECTION('ref_axis',(-9.91270557701033E-17,0.,-1.));
#6670=DIRECTION('',(0.,-1.,0.));
#6671=DIRECTION('center_axis',(0.,-1.,0.));
#6672=DIRECTION('ref_axis',(1.22464679914735E-16,0.,1.));
#6673=DIRECTION('',(0.,-1.,0.));
#6674=DIRECTION('center_axis',(-1.,0.,0.));
#6675=DIRECTION('ref_axis',(0.,0.,1.));
#6676=DIRECTION('',(0.,-1.,0.));
#6677=DIRECTION('center_axis',(0.,-1.,0.));
#6678=DIRECTION('ref_axis',(0.,0.,-1.));
#6679=DIRECTION('',(0.,-1.,0.));
#6680=DIRECTION('center_axis',(0.,0.,-1.));
#6681=DIRECTION('ref_axis',(-1.,0.,0.));
#6682=DIRECTION('',(0.,-1.,0.));
#6683=DIRECTION('center_axis',(-0.707106781186519,0.,-0.707106781186576));
#6684=DIRECTION('ref_axis',(-0.707106781186576,0.,0.707106781186519));
#6685=DIRECTION('',(0.,-1.,0.));
#6686=DIRECTION('center_axis',(-0.707106781186546,0.,0.707106781186549));
#6687=DIRECTION('ref_axis',(0.707106781186549,0.,0.707106781186546));
#6688=DIRECTION('',(0.,-1.,0.));
#6689=DIRECTION('center_axis',(-0.707106781186547,0.,-0.707106781186548));
#6690=DIRECTION('ref_axis',(-0.707106781186548,0.,0.707106781186547));
#6691=DIRECTION('',(0.,-1.,0.));
#6692=DIRECTION('center_axis',(-0.707106781186547,0.,0.707106781186548));
#6693=DIRECTION('ref_axis',(0.707106781186548,0.,0.707106781186547));
#6694=DIRECTION('',(0.,-1.,0.));
#6695=DIRECTION('center_axis',(-0.707106781186549,0.,-0.707106781186546));
#6696=DIRECTION('ref_axis',(-0.707106781186546,0.,0.707106781186549));
#6697=DIRECTION('',(0.,-1.,0.));
#6698=DIRECTION('center_axis',(0.,-1.,0.));
#6699=DIRECTION('ref_axis',(0.,0.,-1.));
#6700=DIRECTION('',(0.,-1.,0.));
#6701=DIRECTION('center_axis',(-0.573576436351023,0.,0.819152044289008));
#6702=DIRECTION('ref_axis',(0.819152044289008,0.,0.573576436351023));
#6703=DIRECTION('',(0.,-1.,0.));
#6704=DIRECTION('center_axis',(-0.819152044288981,0.,-0.573576436351062));
#6705=DIRECTION('ref_axis',(-0.573576436351062,0.,0.819152044288981));
#6706=DIRECTION('',(0.,-1.,0.));
#6707=DIRECTION('center_axis',(-0.573576436351053,0.,0.819152044288987));
#6708=DIRECTION('ref_axis',(0.819152044288987,0.,0.573576436351053));
#6709=DIRECTION('',(0.,-1.,0.));
#6710=DIRECTION('center_axis',(-0.819152044288999,0.,-0.573576436351036));
#6711=DIRECTION('ref_axis',(-0.573576436351036,0.,0.819152044288999));
#6712=DIRECTION('',(0.,-1.,0.));
#6713=DIRECTION('center_axis',(-0.57357643635104,0.,0.819152044288996));
#6714=DIRECTION('ref_axis',(0.819152044288996,0.,0.57357643635104));
#6715=DIRECTION('',(0.,-1.,0.));
#6716=DIRECTION('center_axis',(-0.819152044288994,0.,-0.573576436351043));
#6717=DIRECTION('ref_axis',(-0.573576436351043,0.,0.819152044288994));
#6718=DIRECTION('',(0.,-1.,0.));
#6719=DIRECTION('center_axis',(-0.984807753012207,0.,0.173648177666936));
#6720=DIRECTION('ref_axis',(0.173648177666936,0.,0.984807753012207));
#6721=DIRECTION('',(0.,-1.,0.));
#6722=DIRECTION('center_axis',(0.173648177666932,0.,0.984807753012208));
#6723=DIRECTION('ref_axis',(0.984807753012208,0.,-0.173648177666932));
#6724=DIRECTION('center_axis',(-0.5,0.,0.866025403784439));
#6725=DIRECTION('ref_axis',(0.866025403784439,0.,0.5));
#6726=DIRECTION('',(0.,1.,0.));
#6727=DIRECTION('',(0.866025403784439,0.,0.499999999999999));
#6728=DIRECTION('',(0.,1.,0.));
#6729=DIRECTION('center_axis',(-0.866025403784439,0.,-0.5));
#6730=DIRECTION('ref_axis',(-0.5,0.,0.866025403784439));
#6731=DIRECTION('',(-0.5,0.,0.866025403784439));
#6732=DIRECTION('',(0.,1.,0.));
#6733=DIRECTION('center_axis',(-0.173648177666935,0.,-0.984807753012207));
#6734=DIRECTION('ref_axis',(-0.984807753012207,0.,0.173648177666935));
#6735=DIRECTION('',(-0.984807753012207,0.,0.173648177666934));
#6736=DIRECTION('',(0.,1.,0.));
#6737=DIRECTION('center_axis',(0.984807753012207,0.,-0.173648177666936));
#6738=DIRECTION('ref_axis',(-0.173648177666936,0.,-0.984807753012207));
#6739=DIRECTION('',(-0.173648177666936,0.,-0.984807753012207));
#6740=DIRECTION('',(0.,1.,0.));
#6741=DIRECTION('center_axis',(0.,1.,0.));
#6742=DIRECTION('ref_axis',(0.,0.,1.));
#6743=DIRECTION('center_axis',(0.,-1.,0.));
#6744=DIRECTION('ref_axis',(0.,0.,1.));
#6745=DIRECTION('center_axis',(0.,1.,0.));
#6746=DIRECTION('ref_axis',(0.,0.,1.));
#6747=DIRECTION('center_axis',(0.,0.,1.));
#6748=DIRECTION('ref_axis',(1.,0.,0.));
#6749=DIRECTION('',(0.,1.,0.));
#6750=DIRECTION('',(1.,0.,0.));
#6751=DIRECTION('',(0.,1.,0.));
#6752=DIRECTION('center_axis',(-1.,0.,7.41956747162227E-17));
#6753=DIRECTION('ref_axis',(7.41956747162227E-17,0.,1.));
#6754=DIRECTION('',(7.41956747162227E-17,0.,1.));
#6755=DIRECTION('',(0.,1.,0.));
#6756=DIRECTION('center_axis',(0.5,0.,-0.866025403784438));
#6757=DIRECTION('ref_axis',(-0.866025403784438,0.,-0.5));
#6758=DIRECTION('',(-0.866025403784438,0.,-0.5));
#6759=DIRECTION('',(0.,1.,0.));
#6760=DIRECTION('center_axis',(0.,1.,0.));
#6761=DIRECTION('ref_axis',(0.,0.,1.));
#6762=DIRECTION('center_axis',(0.,-1.,0.));
#6763=DIRECTION('ref_axis',(0.,0.,1.));
#6764=DIRECTION('',(0.,1.,0.));
#6765=DIRECTION('center_axis',(1.,0.,-5.78241158658935E-16));
#6766=DIRECTION('ref_axis',(-5.78241158658935E-16,0.,-1.));
#6767=DIRECTION('',(-5.78241158658935E-16,0.,-1.));
#6768=DIRECTION('center_axis',(0.,1.,0.));
#6769=DIRECTION('ref_axis',(0.,0.,1.));
#6770=DIRECTION('center_axis',(0.,1.,0.));
#6771=DIRECTION('ref_axis',(1.22464679914735E-16,0.,-1.));
#6772=DIRECTION('',(0.,1.,0.));
#6773=DIRECTION('center_axis',(0.,-1.,0.));
#6774=DIRECTION('ref_axis',(0.,0.,1.));
#6775=DIRECTION('',(0.,1.,0.));
#6776=DIRECTION('center_axis',(0.,0.,1.));
#6777=DIRECTION('ref_axis',(1.,0.,0.));
#6778=DIRECTION('',(1.,0.,0.));
#6779=DIRECTION('',(0.,1.,0.));
#6780=DIRECTION('center_axis',(-1.,0.,4.45418905079446E-17));
#6781=DIRECTION('ref_axis',(4.45418905079446E-17,0.,1.));
#6782=DIRECTION('',(4.45418905079446E-17,0.,1.));
#6783=DIRECTION('',(0.,1.,0.));
#6784=DIRECTION('center_axis',(0.,0.,-1.));
#6785=DIRECTION('ref_axis',(-1.,0.,0.));
#6786=DIRECTION('',(-1.,0.,0.));
#6787=DIRECTION('',(0.,1.,0.));
#6788=DIRECTION('center_axis',(1.,0.,0.));
#6789=DIRECTION('ref_axis',(0.,0.,-1.));
#6790=DIRECTION('',(0.,0.,-1.));
#6791=DIRECTION('',(0.,1.,0.));
#6792=DIRECTION('center_axis',(0.,1.,0.));
#6793=DIRECTION('ref_axis',(0.,0.,1.));
#6794=DIRECTION('center_axis',(0.,-1.,0.));
#6795=DIRECTION('ref_axis',(0.,0.,1.));
#6796=DIRECTION('',(0.,1.,0.));
#6797=DIRECTION('center_axis',(1.,0.,8.19364478113207E-17));
#6798=DIRECTION('ref_axis',(8.19364478113207E-17,0.,-1.));
#6799=DIRECTION('',(8.19364478113207E-17,0.,-1.));
#6800=DIRECTION('',(0.,1.,0.));
#6801=DIRECTION('center_axis',(0.,0.,1.));
#6802=DIRECTION('ref_axis',(1.,0.,0.));
#6803=DIRECTION('',(1.,0.,0.));
#6804=DIRECTION('center_axis',(0.,1.,0.));
#6805=DIRECTION('ref_axis',(0.,0.,1.));
#6806=DIRECTION('center_axis',(-4.33680868994201E-16,0.,1.));
#6807=DIRECTION('ref_axis',(1.,0.,4.33680868994201E-16));
#6808=DIRECTION('',(-1.,0.,-4.33680868994201E-16));
#6809=DIRECTION('',(0.,-1.,0.));
#6810=DIRECTION('center_axis',(1.,0.,8.19364478113207E-17));
#6811=DIRECTION('ref_axis',(8.19364478113207E-17,0.,-1.));
#6812=DIRECTION('',(-8.19364478113207E-17,0.,1.));
#6813=DIRECTION('',(0.,-1.,0.));
#6814=DIRECTION('center_axis',(0.,-1.,0.));
#6815=DIRECTION('ref_axis',(0.,0.,-1.));
#6816=DIRECTION('center_axis',(0.,1.,0.));
#6817=DIRECTION('ref_axis',(0.,0.,-1.));
#6818=DIRECTION('',(0.,-1.,0.));
#6819=DIRECTION('center_axis',(1.,0.,-2.89120579329468E-16));
#6820=DIRECTION('ref_axis',(-2.89120579329468E-16,0.,-1.));
#6821=DIRECTION('',(2.89120579329468E-16,0.,1.));
#6822=DIRECTION('',(0.,-1.,0.));
#6823=DIRECTION('center_axis',(0.,0.,-1.));
#6824=DIRECTION('ref_axis',(-1.,0.,0.));
#6825=DIRECTION('',(1.,0.,0.));
#6826=DIRECTION('',(0.,-1.,0.));
#6827=DIRECTION('center_axis',(-1.,0.,4.45418905079446E-17));
#6828=DIRECTION('ref_axis',(4.45418905079446E-17,0.,1.));
#6829=DIRECTION('',(-4.45418905079446E-17,0.,-1.));
#6830=DIRECTION('',(0.,-1.,0.));
#6831=DIRECTION('center_axis',(0.,0.,1.));
#6832=DIRECTION('ref_axis',(1.,0.,0.));
#6833=DIRECTION('',(-1.,0.,0.));
#6834=DIRECTION('center_axis',(0.,-1.,0.));
#6835=DIRECTION('ref_axis',(0.,0.,-1.));
#6836=DIRECTION('center_axis',(-0.866025403784439,0.,-0.5));
#6837=DIRECTION('ref_axis',(-0.5,0.,0.866025403784439));
#6838=DIRECTION('',(0.,-1.,0.));
#6839=DIRECTION('',(0.5,0.,-0.866025403784439));
#6840=DIRECTION('',(0.,-1.,0.));
#6841=DIRECTION('center_axis',(-0.5,0.,0.866025403784439));
#6842=DIRECTION('ref_axis',(0.866025403784439,0.,0.5));
#6843=DIRECTION('',(-0.866025403784439,0.,-0.499999999999999));
#6844=DIRECTION('',(0.,-1.,0.));
#6845=DIRECTION('center_axis',(0.,-1.,0.));
#6846=DIRECTION('ref_axis',(0.,0.,-1.));
#6847=DIRECTION('center_axis',(0.,1.,0.));
#6848=DIRECTION('ref_axis',(0.,0.,-1.));
#6849=DIRECTION('',(0.,-1.,0.));
#6850=DIRECTION('center_axis',(0.984807753012207,0.,-0.173648177666936));
#6851=DIRECTION('ref_axis',(-0.173648177666936,0.,-0.984807753012207));
#6852=DIRECTION('',(0.173648177666936,0.,0.984807753012207));
#6853=DIRECTION('',(0.,-1.,0.));
#6854=DIRECTION('center_axis',(-0.173648177666935,0.,-0.984807753012207));
#6855=DIRECTION('ref_axis',(-0.984807753012207,0.,0.173648177666935));
#6856=DIRECTION('',(0.984807753012207,0.,-0.173648177666934));
#6857=DIRECTION('center_axis',(0.,-1.,0.));
#6858=DIRECTION('ref_axis',(0.,0.,-1.));
#6859=DIRECTION('center_axis',(-1.,0.,7.41956747162227E-17));
#6860=DIRECTION('ref_axis',(7.41956747162227E-17,0.,1.));
#6861=DIRECTION('',(0.,-1.,0.));
#6862=DIRECTION('',(-7.41956747162227E-17,0.,-1.));
#6863=DIRECTION('',(0.,-1.,0.));
#6864=DIRECTION('center_axis',(0.,0.,1.));
#6865=DIRECTION('ref_axis',(1.,0.,0.));
#6866=DIRECTION('',(-1.,0.,0.));
#6867=DIRECTION('',(0.,-1.,0.));
#6868=DIRECTION('center_axis',(1.,0.,-5.20417042793039E-15));
#6869=DIRECTION('ref_axis',(-5.20417042793039E-15,0.,-1.));
#6870=DIRECTION('',(5.20417042793039E-15,0.,1.));
#6871=DIRECTION('',(0.,-1.,0.));
#6872=DIRECTION('center_axis',(0.,-1.,0.));
#6873=DIRECTION('ref_axis',(0.,0.,-1.));
#6874=DIRECTION('center_axis',(0.,1.,0.));
#6875=DIRECTION('ref_axis',(0.,0.,-1.));
#6876=DIRECTION('',(0.,-1.,0.));
#6877=DIRECTION('center_axis',(0.5,0.,-0.866025403784438));
#6878=DIRECTION('ref_axis',(-0.866025403784438,0.,-0.5));
#6879=DIRECTION('',(0.866025403784438,0.,0.5));
#6880=DIRECTION('center_axis',(0.,-1.,0.));
#6881=DIRECTION('ref_axis',(0.,0.,-1.));
#8065=CARTESIAN_POINT('',(0.,0.,0.));
#8066=CARTESIAN_POINT('Origin',(0.,1.,-30.));
#8067=CARTESIAN_POINT('',(-4.28626379701573E-16,0.,-26.5));
#8068=CARTESIAN_POINT('Origin',(0.,0.,-30.));
#8069=CARTESIAN_POINT('',(-4.28626379701573E-16,1.,-26.5));
#8070=CARTESIAN_POINT('',(-4.28626379701573E-16,1.,-26.5));
#8071=CARTESIAN_POINT('Origin',(0.,1.,-30.));
#8072=CARTESIAN_POINT('Origin',(0.,1.,-7.86046575051991E-16));
#8073=CARTESIAN_POINT('',(3.50000000000001,1.,-2.82842712474618));
#8074=CARTESIAN_POINT('',(-3.50000000000001,1.,-2.82842712474618));
#8075=CARTESIAN_POINT('Origin',(0.,1.,-7.86046575051991E-16));
#8076=CARTESIAN_POINT('',(3.50000000000001,0.,-2.82842712474618));
#8077=CARTESIAN_POINT('',(3.50000000000001,1.,-2.82842712474618));
#8078=CARTESIAN_POINT('',(-3.50000000000001,0.,-2.82842712474618));
#8079=CARTESIAN_POINT('Origin',(0.,0.,-7.86046575051991E-16));
#8080=CARTESIAN_POINT('',(-3.50000000000001,1.,-2.82842712474618));
#8081=CARTESIAN_POINT('Origin',(0.,7.,-30.));
#8082=CARTESIAN_POINT('',(-4.28626379701574E-16,8.,-33.5));
#8083=CARTESIAN_POINT('Origin',(0.,8.,-30.));
#8084=CARTESIAN_POINT('',(-4.28626379701574E-16,7.,-33.5));
#8085=CARTESIAN_POINT('',(-4.28626379701574E-16,7.,-33.5));
#8086=CARTESIAN_POINT('Origin',(0.,7.,-30.));
#8087=CARTESIAN_POINT('Origin',(0.,8.,-30.));
#8088=CARTESIAN_POINT('',(-3.06161699786839E-16,8.,-27.5));
#8089=CARTESIAN_POINT('Origin',(0.,8.,-30.));
#8090=CARTESIAN_POINT('',(-3.06161699786839E-16,0.,-27.5));
#8091=CARTESIAN_POINT('',(-3.06161699786839E-16,8.,-27.5));
#8092=CARTESIAN_POINT('Origin',(0.,0.,-30.));
#8093=CARTESIAN_POINT('Origin',(0.,8.,-7.86046575051991E-16));
#8094=CARTESIAN_POINT('',(-3.06161699786838E-16,8.,2.5));
#8095=CARTESIAN_POINT('Origin',(0.,8.,-7.86046575051991E-16));
#8096=CARTESIAN_POINT('',(-3.06161699786838E-16,0.,2.5));
#8097=CARTESIAN_POINT('',(-3.06161699786838E-16,8.,2.5));
#8098=CARTESIAN_POINT('Origin',(0.,0.,-7.86046575051991E-16));
#8099=CARTESIAN_POINT('Origin',(0.,0.,-7.86046575051991E-16));
#8100=CARTESIAN_POINT('Origin',(0.,8.,-7.86046575051991E-16));
#8101=CARTESIAN_POINT('Origin',(0.,8.,-7.86046575051991E-16));
#8102=CARTESIAN_POINT('',(6.25000000000002,8.,-92.0836477965032));
#8103=CARTESIAN_POINT('',(-6.50000000000001,8.,-70.));
#8104=CARTESIAN_POINT('',(6.25000000000002,8.,-92.0836477965032));
#8105=CARTESIAN_POINT('',(-6.50000000000001,8.,0.));
#8106=CARTESIAN_POINT('',(-6.50000000000001,8.,-70.));
#8107=CARTESIAN_POINT('',(6.50000000000001,8.,-3.880363653291E-16));
#8108=CARTESIAN_POINT('Origin',(0.,8.,-7.86046575051991E-16));
#8109=CARTESIAN_POINT('',(6.50000000000001,8.,-24.));
#8110=CARTESIAN_POINT('',(6.50000000000001,8.,-7.86046575051991E-16));
#8111=CARTESIAN_POINT('',(16.5,8.,-34.));
#8112=CARTESIAN_POINT('Origin',(16.5,8.,-24.));
#8113=CARTESIAN_POINT('',(19.5,8.,-34.));
#8114=CARTESIAN_POINT('',(16.5,8.,-34.));
#8115=CARTESIAN_POINT('',(21.6213203435597,8.,-36.1213203435596));
#8116=CARTESIAN_POINT('',(19.5,8.,-34.));
#8117=CARTESIAN_POINT('',(19.6213203435597,8.,-38.1213203435595));
#8118=CARTESIAN_POINT('',(21.6213203435597,8.,-36.1213203435596));
#8119=CARTESIAN_POINT('',(21.6213203435597,8.,-40.1213203435595));
#8120=CARTESIAN_POINT('',(19.6213203435597,8.,-38.1213203435595));
#8121=CARTESIAN_POINT('',(19.6213203435597,8.,-42.1213203435595));
#8122=CARTESIAN_POINT('',(21.6213203435597,8.,-40.1213203435595));
#8123=CARTESIAN_POINT('',(21.6213203435597,8.,-44.1213203435596));
#8124=CARTESIAN_POINT('',(19.6213203435597,8.,-42.1213203435595));
#8125=CARTESIAN_POINT('',(13.5356539813314,8.,-79.5585032438718));
#8126=CARTESIAN_POINT('Origin',(31.3216319671078,8.,-64.9756713141856));
#8127=CARTESIAN_POINT('',(11.2187421199729,8.,-81.1808223945624));
#8128=CARTESIAN_POINT('',(13.5356539813313,8.,-79.5585032438719));
#8129=CARTESIAN_POINT('',(12.8410612706636,8.,-83.4977342559207));
#8130=CARTESIAN_POINT('',(11.2187421199729,8.,-81.1808223945624));
#8131=CARTESIAN_POINT('',(10.5241494093054,8.,-85.1200534066112));
#8132=CARTESIAN_POINT('',(12.8410612706636,8.,-83.4977342559207));
#8133=CARTESIAN_POINT('',(12.1464685599959,8.,-87.4369652679695));
#8134=CARTESIAN_POINT('',(10.5241494093054,8.,-85.1200534066112));
#8135=CARTESIAN_POINT('',(9.82955669863762,8.,-89.05928441866));
#8136=CARTESIAN_POINT('',(12.1464685599959,8.,-87.4369652679695));
#8137=CARTESIAN_POINT('',(11.4518758493282,8.,-91.3761962800183));
#8138=CARTESIAN_POINT('',(9.82955669863762,8.,-89.05928441866));
#8139=CARTESIAN_POINT('',(11.1740387650611,8.,-92.9518886848378));
#8140=CARTESIAN_POINT('',(11.4518758493282,8.,-91.3761962800183));
#8141=CARTESIAN_POINT('',(11.1740387650611,8.,-92.9518886848378));
#8142=CARTESIAN_POINT('',(-3.50000000000001,8.,-2.82842712474618));
#8143=CARTESIAN_POINT('',(3.50000000000001,8.,-2.82842712474618));
#8144=CARTESIAN_POINT('Origin',(0.,8.,-7.86046575051991E-16));
#8145=CARTESIAN_POINT('',(-4.50000000000001,8.,-2.82842712474618));
#8146=CARTESIAN_POINT('',(-4.50000000000001,8.,-2.82842712474618));
#8147=CARTESIAN_POINT('',(-4.50000000000001,8.,-41.7743150561845));
#8148=CARTESIAN_POINT('',(-4.50000000000001,8.,-2.82842712474618));
#8149=CARTESIAN_POINT('',(14.1836440347594,8.,-41.7743150561845));
#8150=CARTESIAN_POINT('',(-4.50000000000001,8.,-41.7743150561845));
#8151=CARTESIAN_POINT('',(14.1836440347594,8.,-35.7743150561845));
#8152=CARTESIAN_POINT('',(14.1836440347594,8.,-41.7743150561845));
#8153=CARTESIAN_POINT('',(4.50000000000001,8.,-24.));
#8154=CARTESIAN_POINT('Origin',(16.5,8.,-24.));
#8155=CARTESIAN_POINT('',(4.50000000000001,8.,-2.82842712474618));
#8156=CARTESIAN_POINT('',(4.50000000000001,8.,-2.82842712474618));
#8157=CARTESIAN_POINT('',(3.50000000000001,8.,-2.82842712474618));
#8158=CARTESIAN_POINT('',(-4.50000000000001,8.,-43.7743150561845));
#8159=CARTESIAN_POINT('',(14.1836440347594,8.,-43.7743150561845));
#8160=CARTESIAN_POINT('',(-4.50000000000001,8.,-43.7743150561845));
#8161=CARTESIAN_POINT('',(-4.50000000000001,8.,-67.1547005383792));
#8162=CARTESIAN_POINT('',(-4.50000000000001,8.,-67.1547005383792));
#8163=CARTESIAN_POINT('',(6.6910990889186,8.,-60.6935164668642));
#8164=CARTESIAN_POINT('',(-4.50000000000001,8.,-67.1547005383792));
#8165=CARTESIAN_POINT('',(14.1836440347593,8.,-46.7743150561846));
#8166=CARTESIAN_POINT('Origin',(31.3216319671078,8.,-64.9756713141856));
#8167=CARTESIAN_POINT('',(14.1836440347594,8.,-43.7743150561845));
#8168=CARTESIAN_POINT('',(-4.50000000000001,8.,-69.4641016151377));
#8169=CARTESIAN_POINT('',(6.38628307923174,8.,-63.1789031488688));
#8170=CARTESIAN_POINT('',(-4.50000000000001,8.,-69.4641016151377));
#8171=CARTESIAN_POINT('',(7.5157431494139,8.,-90.2759792406202));
#8172=CARTESIAN_POINT('',(7.5157431494139,8.,-90.2759792406202));
#8173=CARTESIAN_POINT('',(8.5669118613583,8.,-90.4613286458126));
#8174=CARTESIAN_POINT('',(7.5157431494139,8.,-90.2759792406202));
#8175=CARTESIAN_POINT('',(10.5956992404498,8.,-78.9555036669016));
#8176=CARTESIAN_POINT('',(8.5669118613583,8.,-90.4613286458126));
#8177=CARTESIAN_POINT('Origin',(31.3216319671078,8.,-64.9756713141856));
#8178=CARTESIAN_POINT('Origin',(0.,0.,-7.86046575051991E-16));
#8179=CARTESIAN_POINT('',(6.25000000000002,0.,-92.0836477965032));
#8180=CARTESIAN_POINT('',(-6.50000000000001,0.,-70.));
#8181=CARTESIAN_POINT('',(6.25000000000002,0.,-92.0836477965032));
#8182=CARTESIAN_POINT('',(11.1740387650611,0.,-92.9518886848378));
#8183=CARTESIAN_POINT('',(11.1740387650611,0.,-92.9518886848378));
#8184=CARTESIAN_POINT('',(11.4518758493282,0.,-91.3761962800183));
#8185=CARTESIAN_POINT('',(11.4518758493282,0.,-91.3761962800183));
#8186=CARTESIAN_POINT('',(9.82955669863762,0.,-89.05928441866));
#8187=CARTESIAN_POINT('',(9.82955669863762,0.,-89.05928441866));
#8188=CARTESIAN_POINT('',(12.1464685599959,0.,-87.4369652679695));
#8189=CARTESIAN_POINT('',(12.1464685599959,0.,-87.4369652679695));
#8190=CARTESIAN_POINT('',(10.5241494093054,0.,-85.1200534066112));
#8191=CARTESIAN_POINT('',(10.5241494093054,0.,-85.1200534066112));
#8192=CARTESIAN_POINT('',(12.8410612706636,0.,-83.4977342559207));
#8193=CARTESIAN_POINT('',(12.8410612706636,0.,-83.4977342559207));
#8194=CARTESIAN_POINT('',(11.2187421199729,0.,-81.1808223945624));
#8195=CARTESIAN_POINT('',(11.2187421199729,0.,-81.1808223945624));
#8196=CARTESIAN_POINT('',(13.5356539813314,0.,-79.5585032438718));
#8197=CARTESIAN_POINT('',(13.5356539813313,0.,-79.5585032438719));
#8198=CARTESIAN_POINT('',(21.6213203435597,0.,-44.1213203435596));
#8199=CARTESIAN_POINT('Origin',(31.3216319671078,0.,-64.9756713141856));
#8200=CARTESIAN_POINT('',(19.6213203435597,0.,-42.1213203435595));
#8201=CARTESIAN_POINT('',(19.6213203435597,0.,-42.1213203435595));
#8202=CARTESIAN_POINT('',(21.6213203435597,0.,-40.1213203435595));
#8203=CARTESIAN_POINT('',(21.6213203435597,0.,-40.1213203435595));
#8204=CARTESIAN_POINT('',(19.6213203435597,0.,-38.1213203435595));
#8205=CARTESIAN_POINT('',(19.6213203435597,0.,-38.1213203435595));
#8206=CARTESIAN_POINT('',(21.6213203435597,0.,-36.1213203435596));
#8207=CARTESIAN_POINT('',(21.6213203435597,0.,-36.1213203435596));
#8208=CARTESIAN_POINT('',(19.5,0.,-34.));
#8209=CARTESIAN_POINT('',(19.5,0.,-34.));
#8210=CARTESIAN_POINT('',(16.5,0.,-34.));
#8211=CARTESIAN_POINT('',(16.5,0.,-34.));
#8212=CARTESIAN_POINT('',(6.50000000000001,0.,-24.));
#8213=CARTESIAN_POINT('Origin',(16.5,0.,-24.));
#8214=CARTESIAN_POINT('',(6.50000000000001,0.,-3.880363653291E-16));
#8215=CARTESIAN_POINT('',(6.50000000000001,0.,-7.86046575051991E-16));
#8216=CARTESIAN_POINT('',(-6.50000000000001,0.,0.));
#8217=CARTESIAN_POINT('Origin',(0.,0.,-7.86046575051991E-16));
#8218=CARTESIAN_POINT('',(-6.50000000000001,0.,-70.));
#8219=CARTESIAN_POINT('',(-4.50000000000001,0.,-67.1547005383792));
#8220=CARTESIAN_POINT('',(6.6910990889186,0.,-60.6935164668642));
#8221=CARTESIAN_POINT('',(-4.50000000000001,0.,-67.1547005383792));
#8222=CARTESIAN_POINT('',(-4.50000000000001,0.,-43.7743150561845));
#8223=CARTESIAN_POINT('',(-4.50000000000001,0.,-43.7743150561845));
#8224=CARTESIAN_POINT('',(14.1836440347594,0.,-43.7743150561845));
#8225=CARTESIAN_POINT('',(14.1836440347594,0.,-43.7743150561845));
#8226=CARTESIAN_POINT('',(14.1836440347593,0.,-46.7743150561846));
#8227=CARTESIAN_POINT('',(14.1836440347593,0.,-46.7743150561846));
#8228=CARTESIAN_POINT('Origin',(31.3216319671078,0.,-64.9756713141856));
#8229=CARTESIAN_POINT('',(7.5157431494139,0.,-90.2759792406203));
#8230=CARTESIAN_POINT('',(8.5669118613583,0.,-90.4613286458126));
#8231=CARTESIAN_POINT('',(7.5157431494139,0.,-90.2759792406202));
#8232=CARTESIAN_POINT('',(-4.50000000000001,0.,-69.4641016151377));
#8233=CARTESIAN_POINT('',(-4.50000000000001,0.,-69.4641016151377));
#8234=CARTESIAN_POINT('',(6.38628307923175,0.,-63.1789031488688));
#8235=CARTESIAN_POINT('',(6.38628307923175,0.,-63.1789031488688));
#8236=CARTESIAN_POINT('',(10.5956992404498,0.,-78.9555036669016));
#8237=CARTESIAN_POINT('Origin',(31.3216319671078,0.,-64.9756713141856));
#8238=CARTESIAN_POINT('',(8.5669118613583,0.,-90.4613286458126));
#8239=CARTESIAN_POINT('',(4.50000000000001,0.,-2.82842712474618));
#8240=CARTESIAN_POINT('',(4.50000000000001,0.,-2.82842712474618));
#8241=CARTESIAN_POINT('',(4.50000000000001,0.,-24.));
#8242=CARTESIAN_POINT('',(4.50000000000001,0.,-24.));
#8243=CARTESIAN_POINT('',(14.1836440347594,0.,-35.7743150561845));
#8244=CARTESIAN_POINT('Origin',(16.5,0.,-24.));
#8245=CARTESIAN_POINT('',(14.1836440347594,0.,-41.7743150561845));
#8246=CARTESIAN_POINT('',(14.1836440347594,0.,-41.7743150561845));
#8247=CARTESIAN_POINT('',(-4.50000000000001,0.,-41.7743150561845));
#8248=CARTESIAN_POINT('',(-4.50000000000001,0.,-41.7743150561845));
#8249=CARTESIAN_POINT('',(-4.50000000000001,0.,-2.82842712474618));
#8250=CARTESIAN_POINT('',(-4.50000000000001,0.,-2.82842712474618));
#8251=CARTESIAN_POINT('',(-3.50000000000001,0.,-2.82842712474618));
#8252=CARTESIAN_POINT('Origin',(6.25000000000002,8.,-92.0836477965032));
#8253=CARTESIAN_POINT('',(-6.50000000000001,8.,-70.));
#8254=CARTESIAN_POINT('',(6.25000000000002,8.,-92.0836477965032));
#8255=CARTESIAN_POINT('Origin',(-6.50000000000001,8.,-70.));
#8256=CARTESIAN_POINT('',(-6.50000000000001,8.,0.));
#8257=CARTESIAN_POINT('Origin',(0.,8.,-7.86046575051991E-16));
#8258=CARTESIAN_POINT('',(6.50000000000001,8.,-3.880363653291E-16));
#8259=CARTESIAN_POINT('Origin',(6.50000000000001,8.,-7.86046575051991E-16));
#8260=CARTESIAN_POINT('',(6.50000000000001,8.,-24.));
#8261=CARTESIAN_POINT('Origin',(16.5,8.,-24.));
#8262=CARTESIAN_POINT('',(16.5,8.,-34.));
#8263=CARTESIAN_POINT('Origin',(16.5,8.,-34.));
#8264=CARTESIAN_POINT('',(19.5,8.,-34.));
#8265=CARTESIAN_POINT('Origin',(19.5,8.,-34.));
#8266=CARTESIAN_POINT('',(21.6213203435597,8.,-36.1213203435596));
#8267=CARTESIAN_POINT('Origin',(21.6213203435597,8.,-36.1213203435596));
#8268=CARTESIAN_POINT('',(19.6213203435597,8.,-38.1213203435595));
#8269=CARTESIAN_POINT('Origin',(19.6213203435597,8.,-38.1213203435595));
#8270=CARTESIAN_POINT('',(21.6213203435597,8.,-40.1213203435595));
#8271=CARTESIAN_POINT('Origin',(21.6213203435597,8.,-40.1213203435595));
#8272=CARTESIAN_POINT('',(19.6213203435597,8.,-42.1213203435595));
#8273=CARTESIAN_POINT('Origin',(19.6213203435597,8.,-42.1213203435595));
#8274=CARTESIAN_POINT('',(21.6213203435597,8.,-44.1213203435596));
#8275=CARTESIAN_POINT('Origin',(31.3216319671078,8.,-64.9756713141856));
#8276=CARTESIAN_POINT('',(13.5356539813314,8.,-79.5585032438718));
#8277=CARTESIAN_POINT('Origin',(13.5356539813313,8.,-79.5585032438719));
#8278=CARTESIAN_POINT('',(11.2187421199729,8.,-81.1808223945624));
#8279=CARTESIAN_POINT('Origin',(11.2187421199729,8.,-81.1808223945624));
#8280=CARTESIAN_POINT('',(12.8410612706636,8.,-83.4977342559207));
#8281=CARTESIAN_POINT('Origin',(12.8410612706636,8.,-83.4977342559207));
#8282=CARTESIAN_POINT('',(10.5241494093054,8.,-85.1200534066112));
#8283=CARTESIAN_POINT('Origin',(10.5241494093054,8.,-85.1200534066112));
#8284=CARTESIAN_POINT('',(12.1464685599959,8.,-87.4369652679695));
#8285=CARTESIAN_POINT('Origin',(12.1464685599959,8.,-87.4369652679695));
#8286=CARTESIAN_POINT('',(9.82955669863762,8.,-89.05928441866));
#8287=CARTESIAN_POINT('Origin',(9.82955669863762,8.,-89.05928441866));
#8288=CARTESIAN_POINT('',(11.4518758493282,8.,-91.3761962800183));
#8289=CARTESIAN_POINT('Origin',(11.4518758493282,8.,-91.3761962800183));
#8290=CARTESIAN_POINT('',(11.1740387650611,8.,-92.9518886848378));
#8291=CARTESIAN_POINT('Origin',(11.1740387650611,8.,-92.9518886848378));
#8292=CARTESIAN_POINT('Origin',(-4.50000000000001,7.,-69.4641016151377));
#8293=CARTESIAN_POINT('',(6.38628307923175,7.,-63.1789031488688));
#8294=CARTESIAN_POINT('',(6.38628307923175,7.,-63.1789031488688));
#8295=CARTESIAN_POINT('',(-4.50000000000001,7.,-69.4641016151377));
#8296=CARTESIAN_POINT('',(-4.50000000000001,7.,-69.4641016151377));
#8297=CARTESIAN_POINT('',(-4.50000000000001,7.,-69.4641016151377));
#8298=CARTESIAN_POINT('Origin',(7.5157431494139,7.,-90.2759792406202));
#8299=CARTESIAN_POINT('',(7.5157431494139,7.,-90.2759792406202));
#8300=CARTESIAN_POINT('',(7.5157431494139,7.,-90.2759792406202));
#8301=CARTESIAN_POINT('',(7.5157431494139,7.,-90.2759792406202));
#8302=CARTESIAN_POINT('Origin',(7.5157431494139,7.,-90.2759792406202));
#8303=CARTESIAN_POINT('',(8.5669118613583,7.,-90.4613286458126));
#8304=CARTESIAN_POINT('',(7.5157431494139,7.,-90.2759792406202));
#8305=CARTESIAN_POINT('',(8.5669118613583,7.,-90.4613286458126));
#8306=CARTESIAN_POINT('Origin',(8.5669118613583,7.,-90.4613286458126));
#8307=CARTESIAN_POINT('',(10.5956992404498,7.,-78.9555036669016));
#8308=CARTESIAN_POINT('',(8.5669118613583,7.,-90.4613286458126));
#8309=CARTESIAN_POINT('',(10.5956992404498,7.,-78.9555036669016));
#8310=CARTESIAN_POINT('Origin',(31.3216319671078,7.,-64.9756713141856));
#8311=CARTESIAN_POINT('Origin',(31.3216319671078,7.,-64.9756713141856));
#8312=CARTESIAN_POINT('Origin',(31.3216319671078,7.,-64.9756713141856));
#8313=CARTESIAN_POINT('Origin',(-4.50000000000001,7.,-43.7743150561845));
#8314=CARTESIAN_POINT('',(14.1836440347594,7.,-43.7743150561845));
#8315=CARTESIAN_POINT('',(14.1836440347594,7.,-43.7743150561845));
#8316=CARTESIAN_POINT('',(-4.50000000000001,7.,-43.7743150561845));
#8317=CARTESIAN_POINT('',(-4.50000000000001,7.,-43.7743150561845));
#8318=CARTESIAN_POINT('',(-4.50000000000001,7.,-43.7743150561845));
#8319=CARTESIAN_POINT('Origin',(-4.50000000000001,7.,-67.1547005383792));
#8320=CARTESIAN_POINT('',(-4.50000000000001,7.,-67.1547005383792));
#8321=CARTESIAN_POINT('',(-4.50000000000001,7.,-67.1547005383792));
#8322=CARTESIAN_POINT('',(-4.50000000000001,7.,-67.1547005383792));
#8323=CARTESIAN_POINT('Origin',(-4.50000000000001,7.,-67.1547005383792));
#8324=CARTESIAN_POINT('',(6.6910990889186,7.,-60.6935164668642));
#8325=CARTESIAN_POINT('',(-4.50000000000001,7.,-67.1547005383792));
#8326=CARTESIAN_POINT('',(6.6910990889186,7.,-60.6935164668642));
#8327=CARTESIAN_POINT('Origin',(31.3216319671078,7.,-64.9756713141856));
#8328=CARTESIAN_POINT('',(14.1836440347593,7.,-46.7743150561846));
#8329=CARTESIAN_POINT('Origin',(31.3216319671078,7.,-64.9756713141856));
#8330=CARTESIAN_POINT('',(14.1836440347593,7.,-46.7743150561846));
#8331=CARTESIAN_POINT('Origin',(14.1836440347594,7.,-43.7743150561845));
#8332=CARTESIAN_POINT('',(14.1836440347594,7.,-43.7743150561845));
#8333=CARTESIAN_POINT('Origin',(31.3216319671078,7.,-64.9756713141856));
#8334=CARTESIAN_POINT('Origin',(0.,7.,-7.86046575051991E-16));
#8335=CARTESIAN_POINT('',(3.50000000000001,7.,-2.82842712474618));
#8336=CARTESIAN_POINT('',(3.50000000000001,7.,-2.82842712474618));
#8337=CARTESIAN_POINT('',(-3.50000000000001,7.,-2.82842712474618));
#8338=CARTESIAN_POINT('Origin',(0.,7.,-7.86046575051991E-16));
#8339=CARTESIAN_POINT('',(-3.50000000000001,7.,-2.82842712474618));
#8340=CARTESIAN_POINT('Origin',(-4.50000000000001,7.,-2.82842712474618));
#8341=CARTESIAN_POINT('',(-4.50000000000001,7.,-2.82842712474618));
#8342=CARTESIAN_POINT('',(-4.50000000000001,7.,-2.82842712474618));
#8343=CARTESIAN_POINT('',(-4.50000000000001,7.,-2.82842712474618));
#8344=CARTESIAN_POINT('Origin',(-4.50000000000001,7.,-2.82842712474618));
#8345=CARTESIAN_POINT('',(-4.50000000000001,7.,-41.7743150561845));
#8346=CARTESIAN_POINT('',(-4.50000000000001,7.,-2.82842712474618));
#8347=CARTESIAN_POINT('',(-4.50000000000001,7.,-41.7743150561845));
#8348=CARTESIAN_POINT('Origin',(-4.50000000000001,7.,-41.7743150561845));
#8349=CARTESIAN_POINT('',(14.1836440347594,7.,-41.7743150561845));
#8350=CARTESIAN_POINT('',(-4.50000000000001,7.,-41.7743150561845));
#8351=CARTESIAN_POINT('',(14.1836440347594,7.,-41.7743150561845));
#8352=CARTESIAN_POINT('Origin',(14.1836440347594,7.,-41.7743150561845));
#8353=CARTESIAN_POINT('',(14.1836440347594,7.,-35.7743150561845));
#8354=CARTESIAN_POINT('',(14.1836440347594,7.,-41.7743150561845));
#8355=CARTESIAN_POINT('',(14.1836440347594,7.,-35.7743150561845));
#8356=CARTESIAN_POINT('Origin',(16.5,7.,-24.));
#8357=CARTESIAN_POINT('',(4.50000000000001,7.,-24.));
#8358=CARTESIAN_POINT('Origin',(16.5,7.,-24.));
#8359=CARTESIAN_POINT('',(4.50000000000001,7.,-24.));
#8360=CARTESIAN_POINT('Origin',(4.50000000000001,7.,-2.82842712474618));
#8361=CARTESIAN_POINT('',(4.50000000000001,7.,-2.82842712474618));
#8362=CARTESIAN_POINT('',(4.50000000000001,7.,-2.82842712474618));
#8363=CARTESIAN_POINT('',(4.50000000000001,7.,-2.82842712474618));
#8364=CARTESIAN_POINT('Origin',(3.50000000000001,7.,-2.82842712474618));
#8365=CARTESIAN_POINT('',(3.50000000000001,7.,-2.82842712474618));
#8366=CARTESIAN_POINT('Origin',(0.,7.,-7.86046575051991E-16));
#8367=CARTESIAN_POINT('Origin',(4.50000000000001,1.,-2.82842712474618));
#8368=CARTESIAN_POINT('',(4.50000000000001,1.,-2.82842712474618));
#8369=CARTESIAN_POINT('',(4.50000000000001,1.,-2.82842712474618));
#8370=CARTESIAN_POINT('',(4.50000000000001,1.,-2.82842712474618));
#8371=CARTESIAN_POINT('Origin',(4.50000000000001,1.,-24.));
#8372=CARTESIAN_POINT('',(4.50000000000001,1.,-24.));
#8373=CARTESIAN_POINT('',(4.50000000000001,1.,-24.));
#8374=CARTESIAN_POINT('',(4.50000000000001,1.,-24.));
#8375=CARTESIAN_POINT('Origin',(16.5,1.,-24.));
#8376=CARTESIAN_POINT('',(14.1836440347594,1.,-35.7743150561845));
#8377=CARTESIAN_POINT('Origin',(16.5,1.,-24.));
#8378=CARTESIAN_POINT('',(14.1836440347594,1.,-35.7743150561845));
#8379=CARTESIAN_POINT('Origin',(14.1836440347594,1.,-41.7743150561845));
#8380=CARTESIAN_POINT('',(14.1836440347594,1.,-41.7743150561845));
#8381=CARTESIAN_POINT('',(14.1836440347594,1.,-41.7743150561845));
#8382=CARTESIAN_POINT('',(14.1836440347594,1.,-41.7743150561845));
#8383=CARTESIAN_POINT('Origin',(-4.50000000000001,1.,-41.7743150561845));
#8384=CARTESIAN_POINT('',(-4.50000000000001,1.,-41.7743150561845));
#8385=CARTESIAN_POINT('',(-4.50000000000001,1.,-41.7743150561845));
#8386=CARTESIAN_POINT('',(-4.50000000000001,1.,-41.7743150561845));
#8387=CARTESIAN_POINT('Origin',(-4.50000000000001,1.,-2.82842712474618));
#8388=CARTESIAN_POINT('',(-4.50000000000001,1.,-2.82842712474618));
#8389=CARTESIAN_POINT('',(-4.50000000000001,1.,-2.82842712474618));
#8390=CARTESIAN_POINT('',(-4.50000000000001,1.,-2.82842712474618));
#8391=CARTESIAN_POINT('Origin',(-3.50000000000001,1.,-2.82842712474618));
#8392=CARTESIAN_POINT('',(-3.50000000000001,1.,-2.82842712474618));
#8393=CARTESIAN_POINT('Origin',(0.,1.,-7.86046575051991E-16));
#8394=CARTESIAN_POINT('Origin',(-4.50000000000001,1.,-69.4641016151377));
#8395=CARTESIAN_POINT('',(7.5157431494139,1.,-90.2759792406202));
#8396=CARTESIAN_POINT('',(7.5157431494139,1.,-90.2759792406202));
#8397=CARTESIAN_POINT('',(-4.50000000000001,1.,-69.4641016151377));
#8398=CARTESIAN_POINT('',(-4.50000000000001,1.,-69.4641016151377));
#8399=CARTESIAN_POINT('',(-4.50000000000001,1.,-69.4641016151377));
#8400=CARTESIAN_POINT('Origin',(6.38628307923175,1.,-63.1789031488688));
#8401=CARTESIAN_POINT('',(6.38628307923175,1.,-63.1789031488688));
#8402=CARTESIAN_POINT('',(6.38628307923175,1.,-63.1789031488688));
#8403=CARTESIAN_POINT('',(6.38628307923175,1.,-63.1789031488688));
#8404=CARTESIAN_POINT('Origin',(31.3216319671078,1.,-64.9756713141856));
#8405=CARTESIAN_POINT('',(10.5956992404498,1.,-78.9555036669016));
#8406=CARTESIAN_POINT('Origin',(31.3216319671078,1.,-64.9756713141856));
#8407=CARTESIAN_POINT('',(10.5956992404498,1.,-78.9555036669016));
#8408=CARTESIAN_POINT('Origin',(8.5669118613583,1.,-90.4613286458126));
#8409=CARTESIAN_POINT('',(8.5669118613583,1.,-90.4613286458126));
#8410=CARTESIAN_POINT('',(8.5669118613583,1.,-90.4613286458126));
#8411=CARTESIAN_POINT('',(8.5669118613583,1.,-90.4613286458126));
#8412=CARTESIAN_POINT('Origin',(7.5157431494139,1.,-90.2759792406202));
#8413=CARTESIAN_POINT('',(7.5157431494139,1.,-90.2759792406202));
#8414=CARTESIAN_POINT('Origin',(31.3216319671078,1.,-64.9756713141856));
#8415=CARTESIAN_POINT('Origin',(-4.50000000000001,1.,-43.7743150561845));
#8416=CARTESIAN_POINT('',(-4.50000000000001,1.,-67.1547005383792));
#8417=CARTESIAN_POINT('',(-4.50000000000001,1.,-67.1547005383792));
#8418=CARTESIAN_POINT('',(-4.50000000000001,1.,-43.7743150561845));
#8419=CARTESIAN_POINT('',(-4.50000000000001,1.,-43.7743150561845));
#8420=CARTESIAN_POINT('',(-4.50000000000001,1.,-43.7743150561845));
#8421=CARTESIAN_POINT('Origin',(14.1836440347594,1.,-43.7743150561845));
#8422=CARTESIAN_POINT('',(14.1836440347594,1.,-43.7743150561845));
#8423=CARTESIAN_POINT('',(14.1836440347594,1.,-43.7743150561845));
#8424=CARTESIAN_POINT('',(14.1836440347594,1.,-43.7743150561845));
#8425=CARTESIAN_POINT('Origin',(14.1836440347593,1.,-46.7743150561846));
#8426=CARTESIAN_POINT('',(14.1836440347593,1.,-46.7743150561846));
#8427=CARTESIAN_POINT('',(14.1836440347593,1.,-46.7743150561846));
#8428=CARTESIAN_POINT('',(14.1836440347593,1.,-46.7743150561846));
#8429=CARTESIAN_POINT('Origin',(31.3216319671078,1.,-64.9756713141856));
#8430=CARTESIAN_POINT('',(6.6910990889186,1.,-60.6935164668642));
#8431=CARTESIAN_POINT('Origin',(31.3216319671078,1.,-64.9756713141856));
#8432=CARTESIAN_POINT('',(6.6910990889186,1.,-60.6935164668642));
#8433=CARTESIAN_POINT('Origin',(-4.50000000000001,1.,-67.1547005383792));
#8434=CARTESIAN_POINT('',(-4.50000000000001,1.,-67.1547005383792));
#8435=CARTESIAN_POINT('Origin',(31.3216319671078,1.,-64.9756713141856));
#12949=UNCERTAINTY_MEASURE_WITH_UNIT(LENGTH_MEASURE(0.01),#12967,
'DISTANCE_ACCURACY_VALUE',
'Maximum model space distance between geometric entities at asserted c
onnectivities');
#12956=UNCERTAINTY_MEASURE_WITH_UNIT(LENGTH_MEASURE(0.01),#12967,
'DISTANCE_ACCURACY_VALUE',
'Maximum model space distance between geometric entities at asserted c
onnectivities');
#12959=(
GEOMETRIC_REPRESENTATION_CONTEXT(3)
GLOBAL_UNCERTAINTY_ASSIGNED_CONTEXT((#12949))
GLOBAL_UNIT_ASSIGNED_CONTEXT((#12967,#12969,#12970))
REPRESENTATION_CONTEXT('','3D')
);
#12966=(
GEOMETRIC_REPRESENTATION_CONTEXT(3)
GLOBAL_UNCERTAINTY_ASSIGNED_CONTEXT((#12956))
GLOBAL_UNIT_ASSIGNED_CONTEXT((#12967,#12969,#12970))
REPRESENTATION_CONTEXT('','3D')
);
#12967=(
LENGTH_UNIT()
NAMED_UNIT(*)
SI_UNIT(.MILLI.,.METRE.)
);
#12969=(
NAMED_UNIT(*)
PLANE_ANGLE_UNIT()
SI_UNIT($,.RADIAN.)
);
#12970=(
NAMED_UNIT(*)
SI_UNIT($,.STERADIAN.)
SOLID_ANGLE_UNIT()
);
#12973=SHAPE_DEFINITION_REPRESENTATION(#12982,#13026);
#12982=PRODUCT_DEFINITION_SHAPE('',$,#13036);
#13026=SHAPE_REPRESENTATION('',(#5783),#12959);
#13033=PRODUCT_DEFINITION_CONTEXT('part definition',#13062,'design');
#13036=PRODUCT_DEFINITION('Cam Grip','Cam Grip',#13045,#13033);
#13045=PRODUCT_DEFINITION_FORMATION('',$,#13066);
#13062=APPLICATION_CONTEXT(
'Core Data for Automotive Mechanical Design Process');
#13063=PRODUCT_CONTEXT('part definition',#13062,'mechanical');
#13066=PRODUCT('Cam Grip','Cam Grip',$,(#13063));
#13075=PRESENTATION_STYLE_ASSIGNMENT((#13080));
#13080=SURFACE_STYLE_USAGE(.BOTH.,#13085);
#13085=SURFACE_SIDE_STYLE('',(#13090));
#13090=SURFACE_STYLE_FILL_AREA(#13095);
#13095=FILL_AREA_STYLE('Opaque(31,36,43)',(#13100));
#13100=FILL_AREA_STYLE_COLOUR('Opaque(31,36,43)',#13105);
#13105=COLOUR_RGB('Opaque(31,36,43)',0.12156862745098,0.141176470588235,
0.168627450980392);
ENDSEC;
END-ISO-10303-21;
